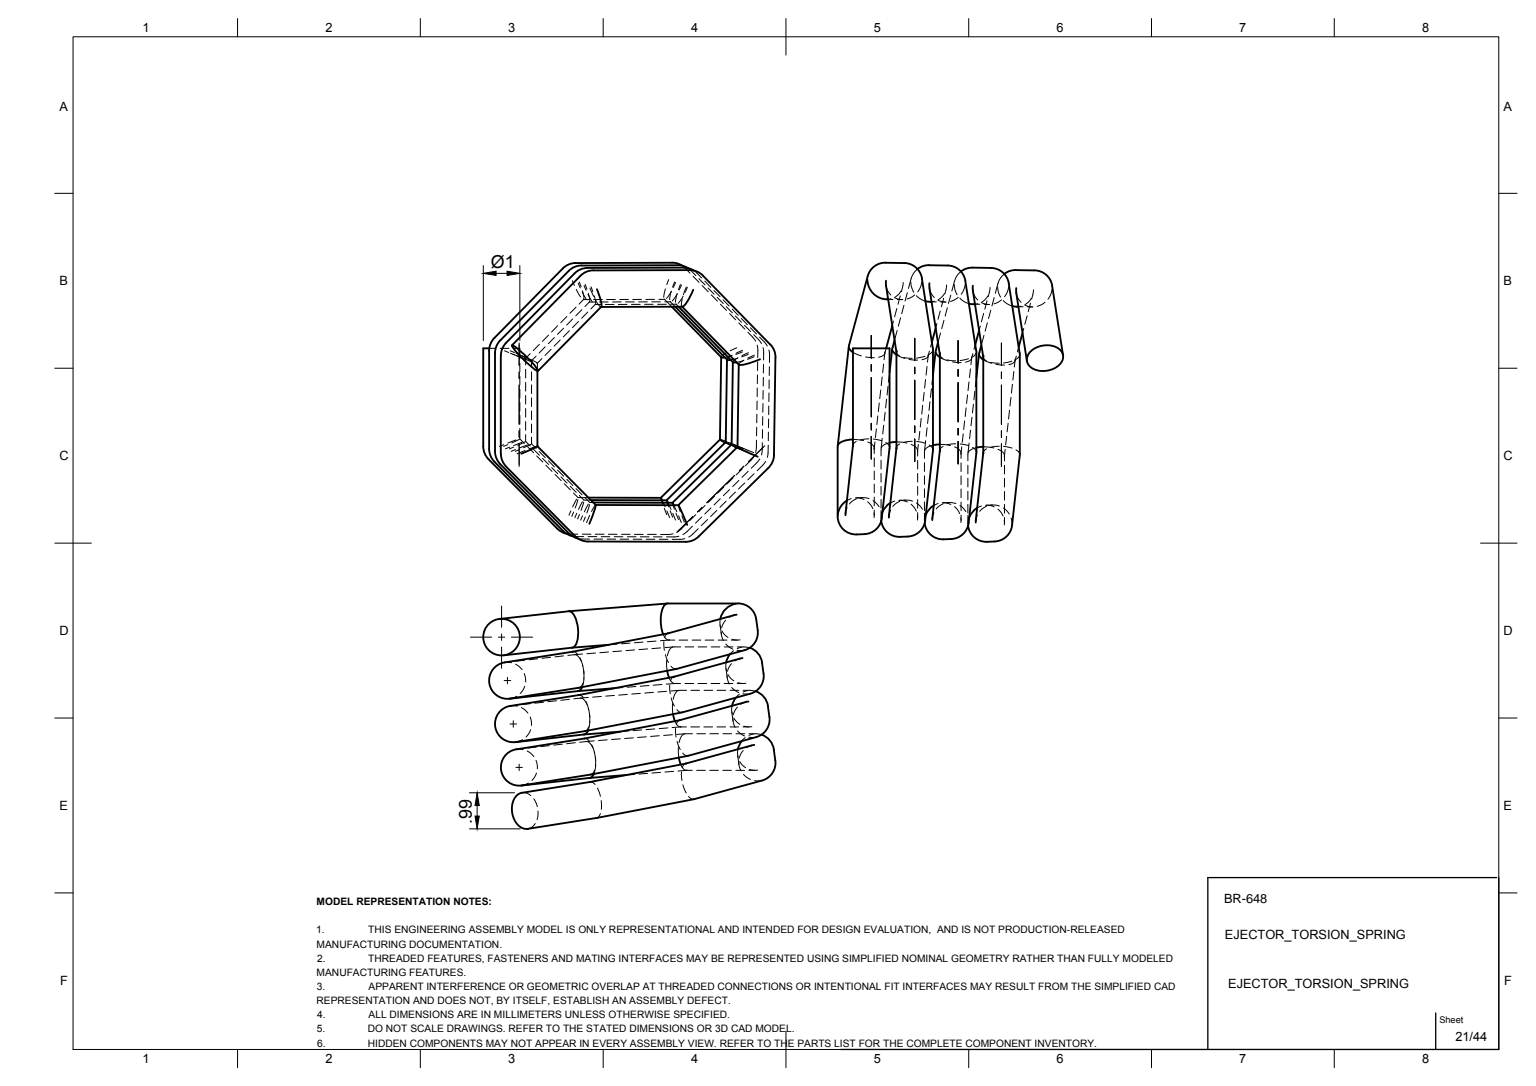
ISO-10303-21;
HEADER;
FILE_DESCRIPTION((''),'2;1');
FILE_NAME('EJECTOR_TORSION_SPRING.step','2026-10-01T22:05:39-07:00',(''),(''),'','','');
FILE_SCHEMA (('AUTOMOTIVE_DESIGN { 1 0 10303 214 3 1 1 }'));
ENDSEC;
DATA;
#10=MECHANICAL_DESIGN_GEOMETRIC_PRESENTATION_REPRESENTATION('',(#621),#24628);
#277=ELLIPSE('',#14403,0.0541051040647724,0.05) ;
#278=ELLIPSE('',#14404,0.0541051040647724,0.05) ;
#279=ELLIPSE('',#14405,0.0541051040647724,0.05) ;
#280=ELLIPSE('',#14408,0.0541051040647731,0.05) ;
#281=ELLIPSE('',#14409,0.0541051040647731,0.05) ;
#282=ELLIPSE('',#14411,0.0541051040647723,0.05) ;
#283=ELLIPSE('',#14413,0.0541051040647739,0.05) ;
#284=ELLIPSE('',#14415,0.0541051040647728,0.05) ;
#285=ELLIPSE('',#14417,0.0541051040647725,0.05) ;
#286=ELLIPSE('',#14418,0.0541051040647725,0.05) ;
#287=ELLIPSE('',#14420,0.0541051040647722,0.05) ;
#288=ELLIPSE('',#14421,0.0541051040647722,0.05) ;
#289=ELLIPSE('',#14422,0.0541051040647722,0.05) ;
#290=ELLIPSE('',#14424,0.0541051040647732,0.05) ;
#291=ELLIPSE('',#14425,0.0541051040647732,0.05) ;
#292=ELLIPSE('',#14427,0.054105104064773,0.05) ;
#293=ELLIPSE('',#14428,0.054105104064773,0.05) ;
#294=ELLIPSE('',#14429,0.054105104064773,0.05) ;
#295=ELLIPSE('',#14431,0.0541051040647731,0.05) ;
#296=ELLIPSE('',#14432,0.0541051040647731,0.05) ;
#297=ELLIPSE('',#14434,0.0541051040647723,0.05) ;
#298=ELLIPSE('',#14436,0.0541051040647739,0.05) ;
#299=ELLIPSE('',#14438,0.0541051040647728,0.05) ;
#300=ELLIPSE('',#14440,0.0541051040647725,0.05) ;
#301=ELLIPSE('',#14441,0.0541051040647725,0.05) ;
#302=ELLIPSE('',#14443,0.0541051040647722,0.05) ;
#303=ELLIPSE('',#14444,0.0541051040647722,0.05) ;
#304=ELLIPSE('',#14445,0.0541051040647722,0.05) ;
#305=ELLIPSE('',#14447,0.0541051040647732,0.05) ;
#306=ELLIPSE('',#14448,0.0541051040647732,0.05) ;
#307=ELLIPSE('',#14450,0.0541051040647732,0.05) ;
#308=ELLIPSE('',#14451,0.0541051040647732,0.05) ;
#309=ELLIPSE('',#14452,0.0541051040647732,0.05) ;
#310=ELLIPSE('',#14454,0.0541051040647731,0.05) ;
#311=ELLIPSE('',#14455,0.0541051040647731,0.05) ;
#312=ELLIPSE('',#14457,0.0541051040647721,0.05) ;
#313=ELLIPSE('',#14459,0.0541051040647739,0.05) ;
#314=ELLIPSE('',#14461,0.0541051040647728,0.05) ;
#315=ELLIPSE('',#14463,0.0541051040647725,0.05) ;
#316=ELLIPSE('',#14464,0.0541051040647725,0.05) ;
#317=ELLIPSE('',#14466,0.0541051040647719,0.05) ;
#318=ELLIPSE('',#14467,0.0541051040647719,0.05) ;
#319=ELLIPSE('',#14468,0.0541051040647719,0.05) ;
#320=ELLIPSE('',#14470,0.0541051040647732,0.05) ;
#321=ELLIPSE('',#14471,0.0541051040647732,0.05) ;
#322=ELLIPSE('',#14473,0.0541051040647732,0.05) ;
#323=ELLIPSE('',#14474,0.0541051040647732,0.05) ;
#324=ELLIPSE('',#14475,0.0541051040647732,0.05) ;
#325=ELLIPSE('',#14477,0.0541051040647731,0.05) ;
#326=ELLIPSE('',#14478,0.0541051040647731,0.05) ;
#327=ELLIPSE('',#14480,0.0541051040647723,0.05) ;
#328=ELLIPSE('',#14482,0.0541051040647732,0.05) ;
#329=ELLIPSE('',#14484,0.0541051040647732,0.05) ;
#330=ELLIPSE('',#14486,0.0541051040647725,0.05) ;
#331=ELLIPSE('',#14487,0.0541051040647725,0.05) ;
#332=ELLIPSE('',#14489,0.0541051040647719,0.05) ;
#333=ELLIPSE('',#14490,0.0541051040647719,0.05) ;
#334=ELLIPSE('',#14491,0.0541051040647719,0.05) ;
#359=SPHERICAL_SURFACE('',#14260,0.05) ;
#360=SPHERICAL_SURFACE('',#14263,0.05) ;
#361=SPHERICAL_SURFACE('',#14269,0.05) ;
#362=SPHERICAL_SURFACE('',#14274,0.05) ;
#363=SPHERICAL_SURFACE('',#14279,0.05) ;
#364=SPHERICAL_SURFACE('',#14284,0.05) ;
#365=SPHERICAL_SURFACE('',#14290,0.05) ;
#366=SPHERICAL_SURFACE('',#14293,0.05) ;
#367=SPHERICAL_SURFACE('',#14296,0.05) ;
#368=SPHERICAL_SURFACE('',#14299,0.05) ;
#369=SPHERICAL_SURFACE('',#14305,0.05) ;
#370=SPHERICAL_SURFACE('',#14310,0.05) ;
#371=SPHERICAL_SURFACE('',#14315,0.05) ;
#372=SPHERICAL_SURFACE('',#14320,0.05) ;
#373=SPHERICAL_SURFACE('',#14326,0.05) ;
#374=SPHERICAL_SURFACE('',#14329,0.05) ;
#375=SPHERICAL_SURFACE('',#14332,0.05) ;
#376=SPHERICAL_SURFACE('',#14335,0.05) ;
#377=SPHERICAL_SURFACE('',#14341,0.05) ;
#378=SPHERICAL_SURFACE('',#14346,0.05) ;
#379=SPHERICAL_SURFACE('',#14351,0.05) ;
#380=SPHERICAL_SURFACE('',#14356,0.05) ;
#381=SPHERICAL_SURFACE('',#14362,0.05) ;
#382=SPHERICAL_SURFACE('',#14365,0.05) ;
#383=SPHERICAL_SURFACE('',#14368,0.05) ;
#384=SPHERICAL_SURFACE('',#14371,0.05) ;
#385=SPHERICAL_SURFACE('',#14377,0.05) ;
#386=SPHERICAL_SURFACE('',#14382,0.05) ;
#387=SPHERICAL_SURFACE('',#14387,0.05) ;
#388=SPHERICAL_SURFACE('',#14392,0.05) ;
#389=SPHERICAL_SURFACE('',#14398,0.05) ;
#537=SHAPE_REPRESENTATION_RELATIONSHIP('SRR','None',#24809,#579) ;
#579=ADVANCED_BREP_SHAPE_REPRESENTATION('',(#661),#24599) ;
#621=STYLED_ITEM('',(#25030),#661) ;
#661=MANIFOLD_SOLID_BREP('EJECTOR_TORSION_SPRING',#13132) ;
#1356=LINE('',#21465,#2192) ;
#1357=LINE('',#21473,#2193) ;
#1358=LINE('',#21477,#2194) ;
#1359=LINE('',#21480,#2195) ;
#1360=LINE('',#21483,#2196) ;
#1361=LINE('',#21486,#2197) ;
#1362=LINE('',#21492,#2198) ;
#1363=LINE('',#21499,#2199) ;
#1364=LINE('',#21504,#2200) ;
#1365=LINE('',#21511,#2201) ;
#1366=LINE('',#21515,#2202) ;
#1367=LINE('',#21518,#2203) ;
#1368=LINE('',#21521,#2204) ;
#1369=LINE('',#21524,#2205) ;
#1370=LINE('',#21530,#2206) ;
#1371=LINE('',#21537,#2207) ;
#1372=LINE('',#21542,#2208) ;
#1373=LINE('',#21549,#2209) ;
#1374=LINE('',#21553,#2210) ;
#1375=LINE('',#21556,#2211) ;
#1376=LINE('',#21559,#2212) ;
#1377=LINE('',#21562,#2213) ;
#1378=LINE('',#21568,#2214) ;
#1379=LINE('',#21575,#2215) ;
#1380=LINE('',#21580,#2216) ;
#1381=LINE('',#21587,#2217) ;
#1382=LINE('',#21591,#2218) ;
#1383=LINE('',#21594,#2219) ;
#1384=LINE('',#21597,#2220) ;
#1385=LINE('',#21600,#2221) ;
#1386=LINE('',#21606,#2222) ;
#1387=LINE('',#21613,#2223) ;
#2192=VECTOR('',#17247,0.05) ;
#2193=VECTOR('',#17258,0.05) ;
#2194=VECTOR('',#17265,0.05) ;
#2195=VECTOR('',#17270,0.05) ;
#2196=VECTOR('',#17275,0.05) ;
#2197=VECTOR('',#17280,0.05) ;
#2198=VECTOR('',#17287,0.05) ;
#2199=VECTOR('',#17296,0.05) ;
#2200=VECTOR('',#17303,0.05) ;
#2201=VECTOR('',#17312,0.05) ;
#2202=VECTOR('',#17319,0.05) ;
#2203=VECTOR('',#17324,0.05) ;
#2204=VECTOR('',#17329,0.05) ;
#2205=VECTOR('',#17334,0.05) ;
#2206=VECTOR('',#17341,0.05) ;
#2207=VECTOR('',#17350,0.05) ;
#2208=VECTOR('',#17357,0.05) ;
#2209=VECTOR('',#17366,0.05) ;
#2210=VECTOR('',#17373,0.05) ;
#2211=VECTOR('',#17378,0.05) ;
#2212=VECTOR('',#17383,0.05) ;
#2213=VECTOR('',#17388,0.05) ;
#2214=VECTOR('',#17395,0.05) ;
#2215=VECTOR('',#17404,0.05) ;
#2216=VECTOR('',#17411,0.05) ;
#2217=VECTOR('',#17420,0.05) ;
#2218=VECTOR('',#17427,0.05) ;
#2219=VECTOR('',#17432,0.05) ;
#2220=VECTOR('',#17437,0.05) ;
#2221=VECTOR('',#17442,0.05) ;
#2222=VECTOR('',#17449,0.05) ;
#2223=VECTOR('',#17458,0.05) ;
#2812=CYLINDRICAL_SURFACE('',#14401,0.05) ;
#2813=CYLINDRICAL_SURFACE('',#14407,0.05) ;
#2814=CYLINDRICAL_SURFACE('',#14410,0.05) ;
#2815=CYLINDRICAL_SURFACE('',#14412,0.05) ;
#2816=CYLINDRICAL_SURFACE('',#14414,0.05) ;
#2817=CYLINDRICAL_SURFACE('',#14416,0.05) ;
#2818=CYLINDRICAL_SURFACE('',#14419,0.05) ;
#2819=CYLINDRICAL_SURFACE('',#14423,0.05) ;
#2820=CYLINDRICAL_SURFACE('',#14426,0.05) ;
#2821=CYLINDRICAL_SURFACE('',#14430,0.05) ;
#2822=CYLINDRICAL_SURFACE('',#14433,0.05) ;
#2823=CYLINDRICAL_SURFACE('',#14435,0.05) ;
#2824=CYLINDRICAL_SURFACE('',#14437,0.05) ;
#2825=CYLINDRICAL_SURFACE('',#14439,0.05) ;
#2826=CYLINDRICAL_SURFACE('',#14442,0.05) ;
#2827=CYLINDRICAL_SURFACE('',#14446,0.05) ;
#2828=CYLINDRICAL_SURFACE('',#14449,0.05) ;
#2829=CYLINDRICAL_SURFACE('',#14453,0.05) ;
#2830=CYLINDRICAL_SURFACE('',#14456,0.05) ;
#2831=CYLINDRICAL_SURFACE('',#14458,0.05) ;
#2832=CYLINDRICAL_SURFACE('',#14460,0.05) ;
#2833=CYLINDRICAL_SURFACE('',#14462,0.05) ;
#2834=CYLINDRICAL_SURFACE('',#14465,0.05) ;
#2835=CYLINDRICAL_SURFACE('',#14469,0.05) ;
#2836=CYLINDRICAL_SURFACE('',#14472,0.05) ;
#2837=CYLINDRICAL_SURFACE('',#14476,0.05) ;
#2838=CYLINDRICAL_SURFACE('',#14479,0.05) ;
#2839=CYLINDRICAL_SURFACE('',#14481,0.05) ;
#2840=CYLINDRICAL_SURFACE('',#14483,0.05) ;
#2841=CYLINDRICAL_SURFACE('',#14485,0.05) ;
#2842=CYLINDRICAL_SURFACE('',#14488,0.05) ;
#2843=CYLINDRICAL_SURFACE('',#14492,0.05) ;
#3244=FACE_OUTER_BOUND('',#4182,.T.) ;
#3245=FACE_OUTER_BOUND('',#4183,.T.) ;
#3246=FACE_OUTER_BOUND('',#4184,.T.) ;
#3247=FACE_OUTER_BOUND('',#4185,.T.) ;
#3248=FACE_OUTER_BOUND('',#4186,.T.) ;
#3249=FACE_OUTER_BOUND('',#4187,.T.) ;
#3250=FACE_OUTER_BOUND('',#4188,.T.) ;
#3251=FACE_OUTER_BOUND('',#4189,.T.) ;
#3252=FACE_OUTER_BOUND('',#4190,.T.) ;
#3253=FACE_OUTER_BOUND('',#4191,.T.) ;
#3254=FACE_OUTER_BOUND('',#4192,.T.) ;
#3255=FACE_OUTER_BOUND('',#4193,.T.) ;
#3256=FACE_OUTER_BOUND('',#4194,.T.) ;
#3257=FACE_OUTER_BOUND('',#4195,.T.) ;
#3258=FACE_OUTER_BOUND('',#4196,.T.) ;
#3259=FACE_OUTER_BOUND('',#4197,.T.) ;
#3260=FACE_OUTER_BOUND('',#4198,.T.) ;
#3261=FACE_OUTER_BOUND('',#4199,.T.) ;
#3262=FACE_OUTER_BOUND('',#4200,.T.) ;
#3263=FACE_OUTER_BOUND('',#4201,.T.) ;
#3264=FACE_OUTER_BOUND('',#4202,.T.) ;
#3265=FACE_OUTER_BOUND('',#4203,.T.) ;
#3266=FACE_OUTER_BOUND('',#4204,.T.) ;
#3267=FACE_OUTER_BOUND('',#4205,.T.) ;
#3268=FACE_OUTER_BOUND('',#4206,.T.) ;
#3269=FACE_OUTER_BOUND('',#4207,.T.) ;
#3270=FACE_OUTER_BOUND('',#4208,.T.) ;
#3271=FACE_OUTER_BOUND('',#4209,.T.) ;
#3272=FACE_OUTER_BOUND('',#4210,.T.) ;
#3273=FACE_OUTER_BOUND('',#4211,.T.) ;
#3274=FACE_OUTER_BOUND('',#4212,.T.) ;
#3275=FACE_OUTER_BOUND('',#4213,.T.) ;
#3276=FACE_OUTER_BOUND('',#4214,.T.) ;
#3277=FACE_OUTER_BOUND('',#4215,.T.) ;
#3278=FACE_OUTER_BOUND('',#4216,.T.) ;
#3279=FACE_OUTER_BOUND('',#4217,.T.) ;
#3280=FACE_OUTER_BOUND('',#4218,.T.) ;
#3281=FACE_OUTER_BOUND('',#4219,.T.) ;
#3282=FACE_OUTER_BOUND('',#4220,.T.) ;
#3283=FACE_OUTER_BOUND('',#4221,.T.) ;
#3284=FACE_OUTER_BOUND('',#4222,.T.) ;
#3285=FACE_OUTER_BOUND('',#4223,.T.) ;
#3286=FACE_OUTER_BOUND('',#4224,.T.) ;
#3287=FACE_OUTER_BOUND('',#4225,.T.) ;
#3288=FACE_OUTER_BOUND('',#4226,.T.) ;
#3289=FACE_OUTER_BOUND('',#4227,.T.) ;
#3290=FACE_OUTER_BOUND('',#4228,.T.) ;
#3291=FACE_OUTER_BOUND('',#4229,.T.) ;
#3292=FACE_OUTER_BOUND('',#4230,.T.) ;
#3293=FACE_OUTER_BOUND('',#4231,.T.) ;
#3294=FACE_OUTER_BOUND('',#4232,.T.) ;
#3295=FACE_OUTER_BOUND('',#4233,.T.) ;
#3296=FACE_OUTER_BOUND('',#4234,.T.) ;
#3297=FACE_OUTER_BOUND('',#4235,.T.) ;
#3298=FACE_OUTER_BOUND('',#4236,.T.) ;
#3299=FACE_OUTER_BOUND('',#4237,.T.) ;
#3300=FACE_OUTER_BOUND('',#4238,.T.) ;
#3301=FACE_OUTER_BOUND('',#4239,.T.) ;
#3302=FACE_OUTER_BOUND('',#4240,.T.) ;
#3303=FACE_OUTER_BOUND('',#4241,.T.) ;
#3304=FACE_OUTER_BOUND('',#4242,.T.) ;
#3305=FACE_OUTER_BOUND('',#4243,.T.) ;
#3306=FACE_OUTER_BOUND('',#4244,.T.) ;
#3307=FACE_OUTER_BOUND('',#4245,.T.) ;
#3308=FACE_OUTER_BOUND('',#4246,.T.) ;
#4182=EDGE_LOOP('',(#9801,#9802)) ;
#4183=EDGE_LOOP('',(#9803,#9804,#9805,#9806,#9807,#9808)) ;
#4184=EDGE_LOOP('',(#9809,#9810,#9811,#9812)) ;
#4185=EDGE_LOOP('',(#9813,#9814,#9815,#9816)) ;
#4186=EDGE_LOOP('',(#9817,#9818,#9819,#9820)) ;
#4187=EDGE_LOOP('',(#9821,#9822,#9823,#9824,#9825,#9826)) ;
#4188=EDGE_LOOP('',(#9827,#9828)) ;
#4189=EDGE_LOOP('',(#9829,#9830)) ;
#4190=EDGE_LOOP('',(#9831,#9832)) ;
#4191=EDGE_LOOP('',(#9833,#9834,#9835,#9836,#9837,#9838)) ;
#4192=EDGE_LOOP('',(#9839,#9840,#9841,#9842)) ;
#4193=EDGE_LOOP('',(#9843,#9844,#9845,#9846)) ;
#4194=EDGE_LOOP('',(#9847,#9848,#9849,#9850)) ;
#4195=EDGE_LOOP('',(#9851,#9852,#9853,#9854,#9855,#9856)) ;
#4196=EDGE_LOOP('',(#9857,#9858)) ;
#4197=EDGE_LOOP('',(#9859,#9860)) ;
#4198=EDGE_LOOP('',(#9861,#9862)) ;
#4199=EDGE_LOOP('',(#9863,#9864,#9865,#9866,#9867,#9868)) ;
#4200=EDGE_LOOP('',(#9869,#9870,#9871,#9872)) ;
#4201=EDGE_LOOP('',(#9873,#9874,#9875,#9876)) ;
#4202=EDGE_LOOP('',(#9877,#9878,#9879,#9880)) ;
#4203=EDGE_LOOP('',(#9881,#9882,#9883,#9884,#9885,#9886)) ;
#4204=EDGE_LOOP('',(#9887,#9888)) ;
#4205=EDGE_LOOP('',(#9889,#9890)) ;
#4206=EDGE_LOOP('',(#9891,#9892)) ;
#4207=EDGE_LOOP('',(#9893,#9894,#9895,#9896,#9897,#9898)) ;
#4208=EDGE_LOOP('',(#9899,#9900,#9901,#9902)) ;
#4209=EDGE_LOOP('',(#9903,#9904,#9905,#9906)) ;
#4210=EDGE_LOOP('',(#9907,#9908,#9909,#9910)) ;
#4211=EDGE_LOOP('',(#9911,#9912,#9913,#9914,#9915,#9916)) ;
#4212=EDGE_LOOP('',(#9917,#9918)) ;
#4213=EDGE_LOOP('',(#9919,#9920,#9921,#9922,#9923,#9924,#9925)) ;
#4214=EDGE_LOOP('',(#9926)) ;
#4215=EDGE_LOOP('',(#9927,#9928,#9929,#9930,#9931,#9932,#9933,#9934,#9935)) ;
#4216=EDGE_LOOP('',(#9936,#9937,#9938,#9939,#9940,#9941,#9942,#9943,#9944,
#9945)) ;
#4217=EDGE_LOOP('',(#9946,#9947,#9948,#9949,#9950,#9951,#9952,#9953)) ;
#4218=EDGE_LOOP('',(#9954,#9955,#9956,#9957,#9958,#9959,#9960,#9961)) ;
#4219=EDGE_LOOP('',(#9962,#9963,#9964,#9965,#9966,#9967,#9968,#9969,#9970,
#9971)) ;
#4220=EDGE_LOOP('',(#9972,#9973,#9974,#9975,#9976,#9977,#9978,#9979,#9980)) ;
#4221=EDGE_LOOP('',(#9981,#9982,#9983,#9984,#9985,#9986,#9987,#9988,#9989)) ;
#4222=EDGE_LOOP('',(#9990,#9991,#9992,#9993,#9994,#9995,#9996,#9997,#9998)) ;
#4223=EDGE_LOOP('',(#9999,#10000,#10001,#10002,#10003,#10004,#10005,#10006,
#10007)) ;
#4224=EDGE_LOOP('',(#10008,#10009,#10010,#10011,#10012,#10013,#10014,#10015,
#10016,#10017)) ;
#4225=EDGE_LOOP('',(#10018,#10019,#10020,#10021,#10022,#10023,#10024,#10025)) ;
#4226=EDGE_LOOP('',(#10026,#10027,#10028,#10029,#10030,#10031,#10032,#10033)) ;
#4227=EDGE_LOOP('',(#10034,#10035,#10036,#10037,#10038,#10039,#10040,#10041,
#10042,#10043)) ;
#4228=EDGE_LOOP('',(#10044,#10045,#10046,#10047,#10048,#10049,#10050,#10051,
#10052)) ;
#4229=EDGE_LOOP('',(#10053,#10054,#10055,#10056,#10057,#10058,#10059,#10060,
#10061)) ;
#4230=EDGE_LOOP('',(#10062,#10063,#10064,#10065,#10066,#10067,#10068,#10069,
#10070)) ;
#4231=EDGE_LOOP('',(#10071,#10072,#10073,#10074,#10075,#10076,#10077,#10078,
#10079)) ;
#4232=EDGE_LOOP('',(#10080,#10081,#10082,#10083,#10084,#10085,#10086,#10087,
#10088,#10089)) ;
#4233=EDGE_LOOP('',(#10090,#10091,#10092,#10093,#10094,#10095,#10096,#10097)) ;
#4234=EDGE_LOOP('',(#10098,#10099,#10100,#10101,#10102,#10103,#10104,#10105)) ;
#4235=EDGE_LOOP('',(#10106,#10107,#10108,#10109,#10110,#10111,#10112,#10113,
#10114,#10115)) ;
#4236=EDGE_LOOP('',(#10116,#10117,#10118,#10119,#10120,#10121,#10122,#10123,
#10124)) ;
#4237=EDGE_LOOP('',(#10125,#10126,#10127,#10128,#10129,#10130,#10131,#10132,
#10133)) ;
#4238=EDGE_LOOP('',(#10134,#10135,#10136,#10137,#10138,#10139,#10140,#10141,
#10142)) ;
#4239=EDGE_LOOP('',(#10143,#10144,#10145,#10146,#10147,#10148,#10149,#10150,
#10151)) ;
#4240=EDGE_LOOP('',(#10152,#10153,#10154,#10155,#10156,#10157,#10158,#10159,
#10160,#10161)) ;
#4241=EDGE_LOOP('',(#10162,#10163,#10164,#10165,#10166,#10167,#10168,#10169)) ;
#4242=EDGE_LOOP('',(#10170,#10171,#10172,#10173,#10174,#10175,#10176,#10177)) ;
#4243=EDGE_LOOP('',(#10178,#10179,#10180,#10181,#10182,#10183,#10184,#10185,
#10186,#10187)) ;
#4244=EDGE_LOOP('',(#10188,#10189,#10190,#10191,#10192,#10193,#10194,#10195,
#10196)) ;
#4245=EDGE_LOOP('',(#10197,#10198,#10199,#10200,#10201,#10202,#10203)) ;
#4246=EDGE_LOOP('',(#10204)) ;
#5048=CIRCLE('',#14261,0.05) ;
#5049=CIRCLE('',#14262,0.05) ;
#5050=CIRCLE('',#14264,0.05) ;
#5051=CIRCLE('',#14265,0.05) ;
#5052=CIRCLE('',#14266,0.05) ;
#5053=CIRCLE('',#14267,0.0499999999999998) ;
#5054=CIRCLE('',#14268,0.05) ;
#5055=CIRCLE('',#14270,0.05) ;
#5056=CIRCLE('',#14271,0.05) ;
#5057=CIRCLE('',#14272,0.05) ;
#5058=CIRCLE('',#14273,0.05) ;
#5059=CIRCLE('',#14275,0.05) ;
#5060=CIRCLE('',#14276,0.05) ;
#5061=CIRCLE('',#14277,0.05) ;
#5062=CIRCLE('',#14278,0.05) ;
#5063=CIRCLE('',#14280,0.05) ;
#5064=CIRCLE('',#14281,0.05) ;
#5065=CIRCLE('',#14282,0.05) ;
#5066=CIRCLE('',#14283,0.05) ;
#5067=CIRCLE('',#14285,0.05) ;
#5068=CIRCLE('',#14286,0.05) ;
#5069=CIRCLE('',#14287,0.0499999999999998) ;
#5070=CIRCLE('',#14288,0.05) ;
#5071=CIRCLE('',#14289,0.05) ;
#5072=CIRCLE('',#14291,0.05) ;
#5073=CIRCLE('',#14292,0.05) ;
#5074=CIRCLE('',#14294,0.05) ;
#5075=CIRCLE('',#14295,0.05) ;
#5076=CIRCLE('',#14297,0.05) ;
#5077=CIRCLE('',#14298,0.05) ;
#5078=CIRCLE('',#14300,0.05) ;
#5079=CIRCLE('',#14301,0.05) ;
#5080=CIRCLE('',#14302,0.05) ;
#5081=CIRCLE('',#14303,0.0499999999999998) ;
#5082=CIRCLE('',#14304,0.05) ;
#5083=CIRCLE('',#14306,0.05) ;
#5084=CIRCLE('',#14307,0.05) ;
#5085=CIRCLE('',#14308,0.05) ;
#5086=CIRCLE('',#14309,0.05) ;
#5087=CIRCLE('',#14311,0.05) ;
#5088=CIRCLE('',#14312,0.05) ;
#5089=CIRCLE('',#14313,0.05) ;
#5090=CIRCLE('',#14314,0.05) ;
#5091=CIRCLE('',#14316,0.05) ;
#5092=CIRCLE('',#14317,0.05) ;
#5093=CIRCLE('',#14318,0.05) ;
#5094=CIRCLE('',#14319,0.05) ;
#5095=CIRCLE('',#14321,0.05) ;
#5096=CIRCLE('',#14322,0.05) ;
#5097=CIRCLE('',#14323,0.0499999999999998) ;
#5098=CIRCLE('',#14324,0.05) ;
#5099=CIRCLE('',#14325,0.05) ;
#5100=CIRCLE('',#14327,0.05) ;
#5101=CIRCLE('',#14328,0.05) ;
#5102=CIRCLE('',#14330,0.05) ;
#5103=CIRCLE('',#14331,0.05) ;
#5104=CIRCLE('',#14333,0.05) ;
#5105=CIRCLE('',#14334,0.05) ;
#5106=CIRCLE('',#14336,0.05) ;
#5107=CIRCLE('',#14337,0.05) ;
#5108=CIRCLE('',#14338,0.05) ;
#5109=CIRCLE('',#14339,0.0499999999999998) ;
#5110=CIRCLE('',#14340,0.05) ;
#5111=CIRCLE('',#14342,0.05) ;
#5112=CIRCLE('',#14343,0.05) ;
#5113=CIRCLE('',#14344,0.05) ;
#5114=CIRCLE('',#14345,0.05) ;
#5115=CIRCLE('',#14347,0.05) ;
#5116=CIRCLE('',#14348,0.05) ;
#5117=CIRCLE('',#14349,0.05) ;
#5118=CIRCLE('',#14350,0.05) ;
#5119=CIRCLE('',#14352,0.05) ;
#5120=CIRCLE('',#14353,0.05) ;
#5121=CIRCLE('',#14354,0.05) ;
#5122=CIRCLE('',#14355,0.05) ;
#5123=CIRCLE('',#14357,0.05) ;
#5124=CIRCLE('',#14358,0.05) ;
#5125=CIRCLE('',#14359,0.0499999999999998) ;
#5126=CIRCLE('',#14360,0.05) ;
#5127=CIRCLE('',#14361,0.05) ;
#5128=CIRCLE('',#14363,0.05) ;
#5129=CIRCLE('',#14364,0.05) ;
#5130=CIRCLE('',#14366,0.05) ;
#5131=CIRCLE('',#14367,0.05) ;
#5132=CIRCLE('',#14369,0.05) ;
#5133=CIRCLE('',#14370,0.05) ;
#5134=CIRCLE('',#14372,0.05) ;
#5135=CIRCLE('',#14373,0.05) ;
#5136=CIRCLE('',#14374,0.05) ;
#5137=CIRCLE('',#14375,0.0499999999999998) ;
#5138=CIRCLE('',#14376,0.05) ;
#5139=CIRCLE('',#14378,0.05) ;
#5140=CIRCLE('',#14379,0.05) ;
#5141=CIRCLE('',#14380,0.05) ;
#5142=CIRCLE('',#14381,0.05) ;
#5143=CIRCLE('',#14383,0.05) ;
#5144=CIRCLE('',#14384,0.05) ;
#5145=CIRCLE('',#14385,0.05) ;
#5146=CIRCLE('',#14386,0.05) ;
#5147=CIRCLE('',#14388,0.05) ;
#5148=CIRCLE('',#14389,0.05) ;
#5149=CIRCLE('',#14390,0.05) ;
#5150=CIRCLE('',#14391,0.05) ;
#5151=CIRCLE('',#14393,0.05) ;
#5152=CIRCLE('',#14394,0.05) ;
#5153=CIRCLE('',#14395,0.0499999999999998) ;
#5154=CIRCLE('',#14396,0.05) ;
#5155=CIRCLE('',#14397,0.05) ;
#5156=CIRCLE('',#14399,0.05) ;
#5157=CIRCLE('',#14400,0.05) ;
#5158=CIRCLE('',#14402,0.05) ;
#5159=CIRCLE('',#14493,0.05) ;
#5975=VERTEX_POINT('',#21211) ;
#5976=VERTEX_POINT('',#21212) ;
#5977=VERTEX_POINT('',#21216) ;
#5978=VERTEX_POINT('',#21217) ;
#5979=VERTEX_POINT('',#21219) ;
#5980=VERTEX_POINT('',#21221) ;
#5981=VERTEX_POINT('',#21223) ;
#5982=VERTEX_POINT('',#21227) ;
#5983=VERTEX_POINT('',#21228) ;
#5984=VERTEX_POINT('',#21230) ;
#5985=VERTEX_POINT('',#21232) ;
#5986=VERTEX_POINT('',#21236) ;
#5987=VERTEX_POINT('',#21237) ;
#5988=VERTEX_POINT('',#21239) ;
#5989=VERTEX_POINT('',#21241) ;
#5990=VERTEX_POINT('',#21245) ;
#5991=VERTEX_POINT('',#21246) ;
#5992=VERTEX_POINT('',#21248) ;
#5993=VERTEX_POINT('',#21250) ;
#5994=VERTEX_POINT('',#21254) ;
#5995=VERTEX_POINT('',#21255) ;
#5996=VERTEX_POINT('',#21257) ;
#5997=VERTEX_POINT('',#21259) ;
#5998=VERTEX_POINT('',#21261) ;
#5999=VERTEX_POINT('',#21265) ;
#6000=VERTEX_POINT('',#21266) ;
#6001=VERTEX_POINT('',#21270) ;
#6002=VERTEX_POINT('',#21271) ;
#6003=VERTEX_POINT('',#21275) ;
#6004=VERTEX_POINT('',#21276) ;
#6005=VERTEX_POINT('',#21280) ;
#6006=VERTEX_POINT('',#21281) ;
#6007=VERTEX_POINT('',#21283) ;
#6008=VERTEX_POINT('',#21285) ;
#6009=VERTEX_POINT('',#21287) ;
#6010=VERTEX_POINT('',#21291) ;
#6011=VERTEX_POINT('',#21292) ;
#6012=VERTEX_POINT('',#21294) ;
#6013=VERTEX_POINT('',#21296) ;
#6014=VERTEX_POINT('',#21300) ;
#6015=VERTEX_POINT('',#21301) ;
#6016=VERTEX_POINT('',#21303) ;
#6017=VERTEX_POINT('',#21305) ;
#6018=VERTEX_POINT('',#21309) ;
#6019=VERTEX_POINT('',#21310) ;
#6020=VERTEX_POINT('',#21312) ;
#6021=VERTEX_POINT('',#21314) ;
#6022=VERTEX_POINT('',#21318) ;
#6023=VERTEX_POINT('',#21319) ;
#6024=VERTEX_POINT('',#21321) ;
#6025=VERTEX_POINT('',#21323) ;
#6026=VERTEX_POINT('',#21325) ;
#6027=VERTEX_POINT('',#21329) ;
#6028=VERTEX_POINT('',#21330) ;
#6029=VERTEX_POINT('',#21334) ;
#6030=VERTEX_POINT('',#21335) ;
#6031=VERTEX_POINT('',#21339) ;
#6032=VERTEX_POINT('',#21340) ;
#6033=VERTEX_POINT('',#21344) ;
#6034=VERTEX_POINT('',#21345) ;
#6035=VERTEX_POINT('',#21347) ;
#6036=VERTEX_POINT('',#21349) ;
#6037=VERTEX_POINT('',#21351) ;
#6038=VERTEX_POINT('',#21355) ;
#6039=VERTEX_POINT('',#21356) ;
#6040=VERTEX_POINT('',#21358) ;
#6041=VERTEX_POINT('',#21360) ;
#6042=VERTEX_POINT('',#21364) ;
#6043=VERTEX_POINT('',#21365) ;
#6044=VERTEX_POINT('',#21367) ;
#6045=VERTEX_POINT('',#21369) ;
#6046=VERTEX_POINT('',#21373) ;
#6047=VERTEX_POINT('',#21374) ;
#6048=VERTEX_POINT('',#21376) ;
#6049=VERTEX_POINT('',#21378) ;
#6050=VERTEX_POINT('',#21382) ;
#6051=VERTEX_POINT('',#21383) ;
#6052=VERTEX_POINT('',#21385) ;
#6053=VERTEX_POINT('',#21387) ;
#6054=VERTEX_POINT('',#21389) ;
#6055=VERTEX_POINT('',#21393) ;
#6056=VERTEX_POINT('',#21394) ;
#6057=VERTEX_POINT('',#21398) ;
#6058=VERTEX_POINT('',#21399) ;
#6059=VERTEX_POINT('',#21403) ;
#6060=VERTEX_POINT('',#21404) ;
#6061=VERTEX_POINT('',#21408) ;
#6062=VERTEX_POINT('',#21409) ;
#6063=VERTEX_POINT('',#21411) ;
#6064=VERTEX_POINT('',#21413) ;
#6065=VERTEX_POINT('',#21415) ;
#6066=VERTEX_POINT('',#21419) ;
#6067=VERTEX_POINT('',#21420) ;
#6068=VERTEX_POINT('',#21422) ;
#6069=VERTEX_POINT('',#21424) ;
#6070=VERTEX_POINT('',#21428) ;
#6071=VERTEX_POINT('',#21429) ;
#6072=VERTEX_POINT('',#21431) ;
#6073=VERTEX_POINT('',#21433) ;
#6074=VERTEX_POINT('',#21437) ;
#6075=VERTEX_POINT('',#21438) ;
#6076=VERTEX_POINT('',#21440) ;
#6077=VERTEX_POINT('',#21442) ;
#6078=VERTEX_POINT('',#21446) ;
#6079=VERTEX_POINT('',#21447) ;
#6080=VERTEX_POINT('',#21449) ;
#6081=VERTEX_POINT('',#21451) ;
#6082=VERTEX_POINT('',#21453) ;
#6083=VERTEX_POINT('',#21457) ;
#6084=VERTEX_POINT('',#21458) ;
#6085=VERTEX_POINT('',#21462) ;
#6086=VERTEX_POINT('',#21464) ;
#6087=VERTEX_POINT('',#21466) ;
#6088=VERTEX_POINT('',#21472) ;
#6089=VERTEX_POINT('',#21487) ;
#6090=VERTEX_POINT('',#21491) ;
#6091=VERTEX_POINT('',#21493) ;
#6092=VERTEX_POINT('',#21498) ;
#6093=VERTEX_POINT('',#21503) ;
#6094=VERTEX_POINT('',#21505) ;
#6095=VERTEX_POINT('',#21510) ;
#6096=VERTEX_POINT('',#21525) ;
#6097=VERTEX_POINT('',#21529) ;
#6098=VERTEX_POINT('',#21531) ;
#6099=VERTEX_POINT('',#21536) ;
#6100=VERTEX_POINT('',#21541) ;
#6101=VERTEX_POINT('',#21543) ;
#6102=VERTEX_POINT('',#21548) ;
#6103=VERTEX_POINT('',#21563) ;
#6104=VERTEX_POINT('',#21567) ;
#6105=VERTEX_POINT('',#21569) ;
#6106=VERTEX_POINT('',#21574) ;
#6107=VERTEX_POINT('',#21579) ;
#6108=VERTEX_POINT('',#21581) ;
#6109=VERTEX_POINT('',#21586) ;
#6110=VERTEX_POINT('',#21601) ;
#6111=VERTEX_POINT('',#21605) ;
#6112=VERTEX_POINT('',#21607) ;
#6113=VERTEX_POINT('',#21612) ;
#7390=EDGE_CURVE('',#5975,#5976,#5048,.T.) ;
#7391=EDGE_CURVE('',#5976,#5975,#5049,.T.) ;
#7392=EDGE_CURVE('',#5977,#5978,#5050,.T.) ;
#7393=EDGE_CURVE('',#5978,#5979,#5051,.T.) ;
#7394=EDGE_CURVE('',#5979,#5980,#5052,.T.) ;
#7395=EDGE_CURVE('',#5981,#5980,#5053,.T.) ;
#7396=EDGE_CURVE('',#5980,#5977,#5054,.T.) ;
#7397=EDGE_CURVE('',#5982,#5983,#5055,.T.) ;
#7398=EDGE_CURVE('',#5983,#5984,#5056,.T.) ;
#7399=EDGE_CURVE('',#5984,#5985,#5057,.T.) ;
#7400=EDGE_CURVE('',#5985,#5982,#5058,.T.) ;
#7401=EDGE_CURVE('',#5986,#5987,#5059,.T.) ;
#7402=EDGE_CURVE('',#5987,#5988,#5060,.T.) ;
#7403=EDGE_CURVE('',#5988,#5989,#5061,.T.) ;
#7404=EDGE_CURVE('',#5989,#5986,#5062,.T.) ;
#7405=EDGE_CURVE('',#5990,#5991,#5063,.T.) ;
#7406=EDGE_CURVE('',#5991,#5992,#5064,.T.) ;
#7407=EDGE_CURVE('',#5992,#5993,#5065,.T.) ;
#7408=EDGE_CURVE('',#5993,#5990,#5066,.T.) ;
#7409=EDGE_CURVE('',#5994,#5995,#5067,.T.) ;
#7410=EDGE_CURVE('',#5995,#5996,#5068,.T.) ;
#7411=EDGE_CURVE('',#5996,#5997,#5069,.T.) ;
#7412=EDGE_CURVE('',#5996,#5998,#5070,.T.) ;
#7413=EDGE_CURVE('',#5998,#5994,#5071,.T.) ;
#7414=EDGE_CURVE('',#5999,#6000,#5072,.T.) ;
#7415=EDGE_CURVE('',#6000,#5999,#5073,.T.) ;
#7416=EDGE_CURVE('',#6001,#6002,#5074,.T.) ;
#7417=EDGE_CURVE('',#6002,#6001,#5075,.T.) ;
#7418=EDGE_CURVE('',#6003,#6004,#5076,.T.) ;
#7419=EDGE_CURVE('',#6004,#6003,#5077,.T.) ;
#7420=EDGE_CURVE('',#6005,#6006,#5078,.T.) ;
#7421=EDGE_CURVE('',#6006,#6007,#5079,.T.) ;
#7422=EDGE_CURVE('',#6007,#6008,#5080,.T.) ;
#7423=EDGE_CURVE('',#6009,#6008,#5081,.T.) ;
#7424=EDGE_CURVE('',#6008,#6005,#5082,.T.) ;
#7425=EDGE_CURVE('',#6010,#6011,#5083,.T.) ;
#7426=EDGE_CURVE('',#6011,#6012,#5084,.T.) ;
#7427=EDGE_CURVE('',#6012,#6013,#5085,.T.) ;
#7428=EDGE_CURVE('',#6013,#6010,#5086,.T.) ;
#7429=EDGE_CURVE('',#6014,#6015,#5087,.T.) ;
#7430=EDGE_CURVE('',#6015,#6016,#5088,.T.) ;
#7431=EDGE_CURVE('',#6016,#6017,#5089,.T.) ;
#7432=EDGE_CURVE('',#6017,#6014,#5090,.T.) ;
#7433=EDGE_CURVE('',#6018,#6019,#5091,.T.) ;
#7434=EDGE_CURVE('',#6019,#6020,#5092,.T.) ;
#7435=EDGE_CURVE('',#6020,#6021,#5093,.T.) ;
#7436=EDGE_CURVE('',#6021,#6018,#5094,.T.) ;
#7437=EDGE_CURVE('',#6022,#6023,#5095,.T.) ;
#7438=EDGE_CURVE('',#6023,#6024,#5096,.T.) ;
#7439=EDGE_CURVE('',#6024,#6025,#5097,.T.) ;
#7440=EDGE_CURVE('',#6024,#6026,#5098,.T.) ;
#7441=EDGE_CURVE('',#6026,#6022,#5099,.T.) ;
#7442=EDGE_CURVE('',#6027,#6028,#5100,.T.) ;
#7443=EDGE_CURVE('',#6028,#6027,#5101,.T.) ;
#7444=EDGE_CURVE('',#6029,#6030,#5102,.T.) ;
#7445=EDGE_CURVE('',#6030,#6029,#5103,.T.) ;
#7446=EDGE_CURVE('',#6031,#6032,#5104,.T.) ;
#7447=EDGE_CURVE('',#6032,#6031,#5105,.T.) ;
#7448=EDGE_CURVE('',#6033,#6034,#5106,.T.) ;
#7449=EDGE_CURVE('',#6034,#6035,#5107,.T.) ;
#7450=EDGE_CURVE('',#6035,#6036,#5108,.T.) ;
#7451=EDGE_CURVE('',#6037,#6036,#5109,.T.) ;
#7452=EDGE_CURVE('',#6036,#6033,#5110,.T.) ;
#7453=EDGE_CURVE('',#6038,#6039,#5111,.T.) ;
#7454=EDGE_CURVE('',#6039,#6040,#5112,.T.) ;
#7455=EDGE_CURVE('',#6040,#6041,#5113,.T.) ;
#7456=EDGE_CURVE('',#6041,#6038,#5114,.T.) ;
#7457=EDGE_CURVE('',#6042,#6043,#5115,.T.) ;
#7458=EDGE_CURVE('',#6043,#6044,#5116,.T.) ;
#7459=EDGE_CURVE('',#6044,#6045,#5117,.T.) ;
#7460=EDGE_CURVE('',#6045,#6042,#5118,.T.) ;
#7461=EDGE_CURVE('',#6046,#6047,#5119,.T.) ;
#7462=EDGE_CURVE('',#6047,#6048,#5120,.T.) ;
#7463=EDGE_CURVE('',#6048,#6049,#5121,.T.) ;
#7464=EDGE_CURVE('',#6049,#6046,#5122,.T.) ;
#7465=EDGE_CURVE('',#6050,#6051,#5123,.T.) ;
#7466=EDGE_CURVE('',#6051,#6052,#5124,.T.) ;
#7467=EDGE_CURVE('',#6052,#6053,#5125,.T.) ;
#7468=EDGE_CURVE('',#6052,#6054,#5126,.T.) ;
#7469=EDGE_CURVE('',#6054,#6050,#5127,.T.) ;
#7470=EDGE_CURVE('',#6055,#6056,#5128,.T.) ;
#7471=EDGE_CURVE('',#6056,#6055,#5129,.T.) ;
#7472=EDGE_CURVE('',#6057,#6058,#5130,.T.) ;
#7473=EDGE_CURVE('',#6058,#6057,#5131,.T.) ;
#7474=EDGE_CURVE('',#6059,#6060,#5132,.T.) ;
#7475=EDGE_CURVE('',#6060,#6059,#5133,.T.) ;
#7476=EDGE_CURVE('',#6061,#6062,#5134,.T.) ;
#7477=EDGE_CURVE('',#6062,#6063,#5135,.T.) ;
#7478=EDGE_CURVE('',#6063,#6064,#5136,.T.) ;
#7479=EDGE_CURVE('',#6065,#6064,#5137,.T.) ;
#7480=EDGE_CURVE('',#6064,#6061,#5138,.T.) ;
#7481=EDGE_CURVE('',#6066,#6067,#5139,.T.) ;
#7482=EDGE_CURVE('',#6067,#6068,#5140,.T.) ;
#7483=EDGE_CURVE('',#6068,#6069,#5141,.T.) ;
#7484=EDGE_CURVE('',#6069,#6066,#5142,.T.) ;
#7485=EDGE_CURVE('',#6070,#6071,#5143,.T.) ;
#7486=EDGE_CURVE('',#6071,#6072,#5144,.T.) ;
#7487=EDGE_CURVE('',#6072,#6073,#5145,.T.) ;
#7488=EDGE_CURVE('',#6073,#6070,#5146,.T.) ;
#7489=EDGE_CURVE('',#6074,#6075,#5147,.T.) ;
#7490=EDGE_CURVE('',#6075,#6076,#5148,.T.) ;
#7491=EDGE_CURVE('',#6076,#6077,#5149,.T.) ;
#7492=EDGE_CURVE('',#6077,#6074,#5150,.T.) ;
#7493=EDGE_CURVE('',#6078,#6079,#5151,.T.) ;
#7494=EDGE_CURVE('',#6079,#6080,#5152,.T.) ;
#7495=EDGE_CURVE('',#6080,#6081,#5153,.T.) ;
#7496=EDGE_CURVE('',#6080,#6082,#5154,.T.) ;
#7497=EDGE_CURVE('',#6082,#6078,#5155,.T.) ;
#7498=EDGE_CURVE('',#6083,#6084,#5156,.T.) ;
#7499=EDGE_CURVE('',#6084,#6083,#5157,.T.) ;
#7500=EDGE_CURVE('',#6085,#6085,#5158,.T.) ;
#7501=EDGE_CURVE('',#6085,#6086,#1356,.T.) ;
#7502=EDGE_CURVE('',#6087,#6086,#277,.T.) ;
#7503=EDGE_CURVE('',#5976,#6087,#278,.T.) ;
#7504=EDGE_CURVE('',#6086,#5975,#279,.T.) ;
#7505=EDGE_CURVE('',#6087,#6088,#1357,.T.) ;
#7506=EDGE_CURVE('',#5978,#6088,#280,.T.) ;
#7507=EDGE_CURVE('',#6088,#5977,#281,.T.) ;
#7508=EDGE_CURVE('',#5979,#5983,#1358,.T.) ;
#7509=EDGE_CURVE('',#5984,#5982,#282,.T.) ;
#7510=EDGE_CURVE('',#5985,#5987,#1359,.T.) ;
#7511=EDGE_CURVE('',#5988,#5986,#283,.T.) ;
#7512=EDGE_CURVE('',#5989,#5991,#1360,.T.) ;
#7513=EDGE_CURVE('',#5992,#5990,#284,.T.) ;
#7514=EDGE_CURVE('',#5993,#5995,#1361,.T.) ;
#7515=EDGE_CURVE('',#6089,#5994,#285,.T.) ;
#7516=EDGE_CURVE('',#5998,#6089,#286,.T.) ;
#7517=EDGE_CURVE('',#6089,#6090,#1362,.T.) ;
#7518=EDGE_CURVE('',#6091,#6090,#287,.T.) ;
#7519=EDGE_CURVE('',#6000,#6091,#288,.T.) ;
#7520=EDGE_CURVE('',#6090,#5999,#289,.T.) ;
#7521=EDGE_CURVE('',#6091,#6092,#1363,.T.) ;
#7522=EDGE_CURVE('',#6002,#6092,#290,.T.) ;
#7523=EDGE_CURVE('',#6092,#6001,#291,.T.) ;
#7524=EDGE_CURVE('',#6092,#6093,#1364,.T.) ;
#7525=EDGE_CURVE('',#6094,#6093,#292,.T.) ;
#7526=EDGE_CURVE('',#6004,#6094,#293,.T.) ;
#7527=EDGE_CURVE('',#6093,#6003,#294,.T.) ;
#7528=EDGE_CURVE('',#6094,#6095,#1365,.T.) ;
#7529=EDGE_CURVE('',#6006,#6095,#295,.T.) ;
#7530=EDGE_CURVE('',#6095,#6005,#296,.T.) ;
#7531=EDGE_CURVE('',#6007,#6011,#1366,.T.) ;
#7532=EDGE_CURVE('',#6012,#6010,#297,.T.) ;
#7533=EDGE_CURVE('',#6013,#6015,#1367,.T.) ;
#7534=EDGE_CURVE('',#6016,#6014,#298,.T.) ;
#7535=EDGE_CURVE('',#6017,#6019,#1368,.T.) ;
#7536=EDGE_CURVE('',#6020,#6018,#299,.T.) ;
#7537=EDGE_CURVE('',#6021,#6023,#1369,.T.) ;
#7538=EDGE_CURVE('',#6096,#6022,#300,.T.) ;
#7539=EDGE_CURVE('',#6026,#6096,#301,.T.) ;
#7540=EDGE_CURVE('',#6096,#6097,#1370,.T.) ;
#7541=EDGE_CURVE('',#6098,#6097,#302,.T.) ;
#7542=EDGE_CURVE('',#6028,#6098,#303,.T.) ;
#7543=EDGE_CURVE('',#6097,#6027,#304,.T.) ;
#7544=EDGE_CURVE('',#6098,#6099,#1371,.T.) ;
#7545=EDGE_CURVE('',#6030,#6099,#305,.T.) ;
#7546=EDGE_CURVE('',#6099,#6029,#306,.T.) ;
#7547=EDGE_CURVE('',#6099,#6100,#1372,.T.) ;
#7548=EDGE_CURVE('',#6101,#6100,#307,.T.) ;
#7549=EDGE_CURVE('',#6032,#6101,#308,.T.) ;
#7550=EDGE_CURVE('',#6100,#6031,#309,.T.) ;
#7551=EDGE_CURVE('',#6101,#6102,#1373,.T.) ;
#7552=EDGE_CURVE('',#6034,#6102,#310,.T.) ;
#7553=EDGE_CURVE('',#6102,#6033,#311,.T.) ;
#7554=EDGE_CURVE('',#6035,#6039,#1374,.T.) ;
#7555=EDGE_CURVE('',#6040,#6038,#312,.T.) ;
#7556=EDGE_CURVE('',#6041,#6043,#1375,.T.) ;
#7557=EDGE_CURVE('',#6044,#6042,#313,.T.) ;
#7558=EDGE_CURVE('',#6045,#6047,#1376,.T.) ;
#7559=EDGE_CURVE('',#6048,#6046,#314,.T.) ;
#7560=EDGE_CURVE('',#6049,#6051,#1377,.T.) ;
#7561=EDGE_CURVE('',#6103,#6050,#315,.T.) ;
#7562=EDGE_CURVE('',#6054,#6103,#316,.T.) ;
#7563=EDGE_CURVE('',#6103,#6104,#1378,.T.) ;
#7564=EDGE_CURVE('',#6105,#6104,#317,.T.) ;
#7565=EDGE_CURVE('',#6056,#6105,#318,.T.) ;
#7566=EDGE_CURVE('',#6104,#6055,#319,.T.) ;
#7567=EDGE_CURVE('',#6105,#6106,#1379,.T.) ;
#7568=EDGE_CURVE('',#6058,#6106,#320,.T.) ;
#7569=EDGE_CURVE('',#6106,#6057,#321,.T.) ;
#7570=EDGE_CURVE('',#6106,#6107,#1380,.T.) ;
#7571=EDGE_CURVE('',#6108,#6107,#322,.T.) ;
#7572=EDGE_CURVE('',#6060,#6108,#323,.T.) ;
#7573=EDGE_CURVE('',#6107,#6059,#324,.T.) ;
#7574=EDGE_CURVE('',#6108,#6109,#1381,.T.) ;
#7575=EDGE_CURVE('',#6062,#6109,#325,.T.) ;
#7576=EDGE_CURVE('',#6109,#6061,#326,.T.) ;
#7577=EDGE_CURVE('',#6063,#6067,#1382,.T.) ;
#7578=EDGE_CURVE('',#6068,#6066,#327,.T.) ;
#7579=EDGE_CURVE('',#6069,#6071,#1383,.T.) ;
#7580=EDGE_CURVE('',#6072,#6070,#328,.T.) ;
#7581=EDGE_CURVE('',#6073,#6075,#1384,.T.) ;
#7582=EDGE_CURVE('',#6076,#6074,#329,.T.) ;
#7583=EDGE_CURVE('',#6077,#6079,#1385,.T.) ;
#7584=EDGE_CURVE('',#6110,#6078,#330,.T.) ;
#7585=EDGE_CURVE('',#6082,#6110,#331,.T.) ;
#7586=EDGE_CURVE('',#6110,#6111,#1386,.T.) ;
#7587=EDGE_CURVE('',#6112,#6111,#332,.T.) ;
#7588=EDGE_CURVE('',#6084,#6112,#333,.T.) ;
#7589=EDGE_CURVE('',#6111,#6083,#334,.T.) ;
#7590=EDGE_CURVE('',#6112,#6113,#1387,.T.) ;
#7591=EDGE_CURVE('',#6113,#6113,#5159,.T.) ;
#9801=ORIENTED_EDGE('',*,*,#7390,.T.) ;
#9802=ORIENTED_EDGE('',*,*,#7391,.T.) ;
#9803=ORIENTED_EDGE('',*,*,#7392,.T.) ;
#9804=ORIENTED_EDGE('',*,*,#7393,.T.) ;
#9805=ORIENTED_EDGE('',*,*,#7394,.T.) ;
#9806=ORIENTED_EDGE('',*,*,#7395,.F.) ;
#9807=ORIENTED_EDGE('',*,*,#7395,.T.) ;
#9808=ORIENTED_EDGE('',*,*,#7396,.T.) ;
#9809=ORIENTED_EDGE('',*,*,#7397,.T.) ;
#9810=ORIENTED_EDGE('',*,*,#7398,.T.) ;
#9811=ORIENTED_EDGE('',*,*,#7399,.T.) ;
#9812=ORIENTED_EDGE('',*,*,#7400,.T.) ;
#9813=ORIENTED_EDGE('',*,*,#7401,.T.) ;
#9814=ORIENTED_EDGE('',*,*,#7402,.T.) ;
#9815=ORIENTED_EDGE('',*,*,#7403,.T.) ;
#9816=ORIENTED_EDGE('',*,*,#7404,.T.) ;
#9817=ORIENTED_EDGE('',*,*,#7405,.T.) ;
#9818=ORIENTED_EDGE('',*,*,#7406,.T.) ;
#9819=ORIENTED_EDGE('',*,*,#7407,.T.) ;
#9820=ORIENTED_EDGE('',*,*,#7408,.T.) ;
#9821=ORIENTED_EDGE('',*,*,#7409,.T.) ;
#9822=ORIENTED_EDGE('',*,*,#7410,.T.) ;
#9823=ORIENTED_EDGE('',*,*,#7411,.T.) ;
#9824=ORIENTED_EDGE('',*,*,#7411,.F.) ;
#9825=ORIENTED_EDGE('',*,*,#7412,.T.) ;
#9826=ORIENTED_EDGE('',*,*,#7413,.T.) ;
#9827=ORIENTED_EDGE('',*,*,#7414,.T.) ;
#9828=ORIENTED_EDGE('',*,*,#7415,.T.) ;
#9829=ORIENTED_EDGE('',*,*,#7416,.T.) ;
#9830=ORIENTED_EDGE('',*,*,#7417,.T.) ;
#9831=ORIENTED_EDGE('',*,*,#7418,.T.) ;
#9832=ORIENTED_EDGE('',*,*,#7419,.T.) ;
#9833=ORIENTED_EDGE('',*,*,#7420,.T.) ;
#9834=ORIENTED_EDGE('',*,*,#7421,.T.) ;
#9835=ORIENTED_EDGE('',*,*,#7422,.T.) ;
#9836=ORIENTED_EDGE('',*,*,#7423,.F.) ;
#9837=ORIENTED_EDGE('',*,*,#7423,.T.) ;
#9838=ORIENTED_EDGE('',*,*,#7424,.T.) ;
#9839=ORIENTED_EDGE('',*,*,#7425,.T.) ;
#9840=ORIENTED_EDGE('',*,*,#7426,.T.) ;
#9841=ORIENTED_EDGE('',*,*,#7427,.T.) ;
#9842=ORIENTED_EDGE('',*,*,#7428,.T.) ;
#9843=ORIENTED_EDGE('',*,*,#7429,.T.) ;
#9844=ORIENTED_EDGE('',*,*,#7430,.T.) ;
#9845=ORIENTED_EDGE('',*,*,#7431,.T.) ;
#9846=ORIENTED_EDGE('',*,*,#7432,.T.) ;
#9847=ORIENTED_EDGE('',*,*,#7433,.T.) ;
#9848=ORIENTED_EDGE('',*,*,#7434,.T.) ;
#9849=ORIENTED_EDGE('',*,*,#7435,.T.) ;
#9850=ORIENTED_EDGE('',*,*,#7436,.T.) ;
#9851=ORIENTED_EDGE('',*,*,#7437,.T.) ;
#9852=ORIENTED_EDGE('',*,*,#7438,.T.) ;
#9853=ORIENTED_EDGE('',*,*,#7439,.T.) ;
#9854=ORIENTED_EDGE('',*,*,#7439,.F.) ;
#9855=ORIENTED_EDGE('',*,*,#7440,.T.) ;
#9856=ORIENTED_EDGE('',*,*,#7441,.T.) ;
#9857=ORIENTED_EDGE('',*,*,#7442,.T.) ;
#9858=ORIENTED_EDGE('',*,*,#7443,.T.) ;
#9859=ORIENTED_EDGE('',*,*,#7444,.T.) ;
#9860=ORIENTED_EDGE('',*,*,#7445,.T.) ;
#9861=ORIENTED_EDGE('',*,*,#7446,.T.) ;
#9862=ORIENTED_EDGE('',*,*,#7447,.T.) ;
#9863=ORIENTED_EDGE('',*,*,#7448,.T.) ;
#9864=ORIENTED_EDGE('',*,*,#7449,.T.) ;
#9865=ORIENTED_EDGE('',*,*,#7450,.T.) ;
#9866=ORIENTED_EDGE('',*,*,#7451,.F.) ;
#9867=ORIENTED_EDGE('',*,*,#7451,.T.) ;
#9868=ORIENTED_EDGE('',*,*,#7452,.T.) ;
#9869=ORIENTED_EDGE('',*,*,#7453,.T.) ;
#9870=ORIENTED_EDGE('',*,*,#7454,.T.) ;
#9871=ORIENTED_EDGE('',*,*,#7455,.T.) ;
#9872=ORIENTED_EDGE('',*,*,#7456,.T.) ;
#9873=ORIENTED_EDGE('',*,*,#7457,.T.) ;
#9874=ORIENTED_EDGE('',*,*,#7458,.T.) ;
#9875=ORIENTED_EDGE('',*,*,#7459,.T.) ;
#9876=ORIENTED_EDGE('',*,*,#7460,.T.) ;
#9877=ORIENTED_EDGE('',*,*,#7461,.T.) ;
#9878=ORIENTED_EDGE('',*,*,#7462,.T.) ;
#9879=ORIENTED_EDGE('',*,*,#7463,.T.) ;
#9880=ORIENTED_EDGE('',*,*,#7464,.T.) ;
#9881=ORIENTED_EDGE('',*,*,#7465,.T.) ;
#9882=ORIENTED_EDGE('',*,*,#7466,.T.) ;
#9883=ORIENTED_EDGE('',*,*,#7467,.T.) ;
#9884=ORIENTED_EDGE('',*,*,#7467,.F.) ;
#9885=ORIENTED_EDGE('',*,*,#7468,.T.) ;
#9886=ORIENTED_EDGE('',*,*,#7469,.T.) ;
#9887=ORIENTED_EDGE('',*,*,#7470,.T.) ;
#9888=ORIENTED_EDGE('',*,*,#7471,.T.) ;
#9889=ORIENTED_EDGE('',*,*,#7472,.T.) ;
#9890=ORIENTED_EDGE('',*,*,#7473,.T.) ;
#9891=ORIENTED_EDGE('',*,*,#7474,.T.) ;
#9892=ORIENTED_EDGE('',*,*,#7475,.T.) ;
#9893=ORIENTED_EDGE('',*,*,#7476,.T.) ;
#9894=ORIENTED_EDGE('',*,*,#7477,.T.) ;
#9895=ORIENTED_EDGE('',*,*,#7478,.T.) ;
#9896=ORIENTED_EDGE('',*,*,#7479,.F.) ;
#9897=ORIENTED_EDGE('',*,*,#7479,.T.) ;
#9898=ORIENTED_EDGE('',*,*,#7480,.T.) ;
#9899=ORIENTED_EDGE('',*,*,#7481,.T.) ;
#9900=ORIENTED_EDGE('',*,*,#7482,.T.) ;
#9901=ORIENTED_EDGE('',*,*,#7483,.T.) ;
#9902=ORIENTED_EDGE('',*,*,#7484,.T.) ;
#9903=ORIENTED_EDGE('',*,*,#7485,.T.) ;
#9904=ORIENTED_EDGE('',*,*,#7486,.T.) ;
#9905=ORIENTED_EDGE('',*,*,#7487,.T.) ;
#9906=ORIENTED_EDGE('',*,*,#7488,.T.) ;
#9907=ORIENTED_EDGE('',*,*,#7489,.T.) ;
#9908=ORIENTED_EDGE('',*,*,#7490,.T.) ;
#9909=ORIENTED_EDGE('',*,*,#7491,.T.) ;
#9910=ORIENTED_EDGE('',*,*,#7492,.T.) ;
#9911=ORIENTED_EDGE('',*,*,#7493,.T.) ;
#9912=ORIENTED_EDGE('',*,*,#7494,.T.) ;
#9913=ORIENTED_EDGE('',*,*,#7495,.T.) ;
#9914=ORIENTED_EDGE('',*,*,#7495,.F.) ;
#9915=ORIENTED_EDGE('',*,*,#7496,.T.) ;
#9916=ORIENTED_EDGE('',*,*,#7497,.T.) ;
#9917=ORIENTED_EDGE('',*,*,#7498,.T.) ;
#9918=ORIENTED_EDGE('',*,*,#7499,.T.) ;
#9919=ORIENTED_EDGE('',*,*,#7500,.F.) ;
#9920=ORIENTED_EDGE('',*,*,#7501,.T.) ;
#9921=ORIENTED_EDGE('',*,*,#7502,.F.) ;
#9922=ORIENTED_EDGE('',*,*,#7503,.F.) ;
#9923=ORIENTED_EDGE('',*,*,#7390,.F.) ;
#9924=ORIENTED_EDGE('',*,*,#7504,.F.) ;
#9925=ORIENTED_EDGE('',*,*,#7501,.F.) ;
#9926=ORIENTED_EDGE('',*,*,#7500,.T.) ;
#9927=ORIENTED_EDGE('',*,*,#7503,.T.) ;
#9928=ORIENTED_EDGE('',*,*,#7505,.T.) ;
#9929=ORIENTED_EDGE('',*,*,#7506,.F.) ;
#9930=ORIENTED_EDGE('',*,*,#7392,.F.) ;
#9931=ORIENTED_EDGE('',*,*,#7507,.F.) ;
#9932=ORIENTED_EDGE('',*,*,#7505,.F.) ;
#9933=ORIENTED_EDGE('',*,*,#7502,.T.) ;
#9934=ORIENTED_EDGE('',*,*,#7504,.T.) ;
#9935=ORIENTED_EDGE('',*,*,#7391,.F.) ;
#9936=ORIENTED_EDGE('',*,*,#7506,.T.) ;
#9937=ORIENTED_EDGE('',*,*,#7507,.T.) ;
#9938=ORIENTED_EDGE('',*,*,#7396,.F.) ;
#9939=ORIENTED_EDGE('',*,*,#7394,.F.) ;
#9940=ORIENTED_EDGE('',*,*,#7508,.T.) ;
#9941=ORIENTED_EDGE('',*,*,#7397,.F.) ;
#9942=ORIENTED_EDGE('',*,*,#7509,.F.) ;
#9943=ORIENTED_EDGE('',*,*,#7398,.F.) ;
#9944=ORIENTED_EDGE('',*,*,#7508,.F.) ;
#9945=ORIENTED_EDGE('',*,*,#7393,.F.) ;
#9946=ORIENTED_EDGE('',*,*,#7509,.T.) ;
#9947=ORIENTED_EDGE('',*,*,#7400,.F.) ;
#9948=ORIENTED_EDGE('',*,*,#7510,.T.) ;
#9949=ORIENTED_EDGE('',*,*,#7401,.F.) ;
#9950=ORIENTED_EDGE('',*,*,#7511,.F.) ;
#9951=ORIENTED_EDGE('',*,*,#7402,.F.) ;
#9952=ORIENTED_EDGE('',*,*,#7510,.F.) ;
#9953=ORIENTED_EDGE('',*,*,#7399,.F.) ;
#9954=ORIENTED_EDGE('',*,*,#7511,.T.) ;
#9955=ORIENTED_EDGE('',*,*,#7404,.F.) ;
#9956=ORIENTED_EDGE('',*,*,#7512,.T.) ;
#9957=ORIENTED_EDGE('',*,*,#7405,.F.) ;
#9958=ORIENTED_EDGE('',*,*,#7513,.F.) ;
#9959=ORIENTED_EDGE('',*,*,#7406,.F.) ;
#9960=ORIENTED_EDGE('',*,*,#7512,.F.) ;
#9961=ORIENTED_EDGE('',*,*,#7403,.F.) ;
#9962=ORIENTED_EDGE('',*,*,#7513,.T.) ;
#9963=ORIENTED_EDGE('',*,*,#7408,.F.) ;
#9964=ORIENTED_EDGE('',*,*,#7514,.T.) ;
#9965=ORIENTED_EDGE('',*,*,#7409,.F.) ;
#9966=ORIENTED_EDGE('',*,*,#7515,.F.) ;
#9967=ORIENTED_EDGE('',*,*,#7516,.F.) ;
#9968=ORIENTED_EDGE('',*,*,#7412,.F.) ;
#9969=ORIENTED_EDGE('',*,*,#7410,.F.) ;
#9970=ORIENTED_EDGE('',*,*,#7514,.F.) ;
#9971=ORIENTED_EDGE('',*,*,#7407,.F.) ;
#9972=ORIENTED_EDGE('',*,*,#7516,.T.) ;
#9973=ORIENTED_EDGE('',*,*,#7517,.T.) ;
#9974=ORIENTED_EDGE('',*,*,#7518,.F.) ;
#9975=ORIENTED_EDGE('',*,*,#7519,.F.) ;
#9976=ORIENTED_EDGE('',*,*,#7414,.F.) ;
#9977=ORIENTED_EDGE('',*,*,#7520,.F.) ;
#9978=ORIENTED_EDGE('',*,*,#7517,.F.) ;
#9979=ORIENTED_EDGE('',*,*,#7515,.T.) ;
#9980=ORIENTED_EDGE('',*,*,#7413,.F.) ;
#9981=ORIENTED_EDGE('',*,*,#7519,.T.) ;
#9982=ORIENTED_EDGE('',*,*,#7521,.T.) ;
#9983=ORIENTED_EDGE('',*,*,#7522,.F.) ;
#9984=ORIENTED_EDGE('',*,*,#7416,.F.) ;
#9985=ORIENTED_EDGE('',*,*,#7523,.F.) ;
#9986=ORIENTED_EDGE('',*,*,#7521,.F.) ;
#9987=ORIENTED_EDGE('',*,*,#7518,.T.) ;
#9988=ORIENTED_EDGE('',*,*,#7520,.T.) ;
#9989=ORIENTED_EDGE('',*,*,#7415,.F.) ;
#9990=ORIENTED_EDGE('',*,*,#7522,.T.) ;
#9991=ORIENTED_EDGE('',*,*,#7524,.T.) ;
#9992=ORIENTED_EDGE('',*,*,#7525,.F.) ;
#9993=ORIENTED_EDGE('',*,*,#7526,.F.) ;
#9994=ORIENTED_EDGE('',*,*,#7418,.F.) ;
#9995=ORIENTED_EDGE('',*,*,#7527,.F.) ;
#9996=ORIENTED_EDGE('',*,*,#7524,.F.) ;
#9997=ORIENTED_EDGE('',*,*,#7523,.T.) ;
#9998=ORIENTED_EDGE('',*,*,#7417,.F.) ;
#9999=ORIENTED_EDGE('',*,*,#7526,.T.) ;
#10000=ORIENTED_EDGE('',*,*,#7528,.T.) ;
#10001=ORIENTED_EDGE('',*,*,#7529,.F.) ;
#10002=ORIENTED_EDGE('',*,*,#7420,.F.) ;
#10003=ORIENTED_EDGE('',*,*,#7530,.F.) ;
#10004=ORIENTED_EDGE('',*,*,#7528,.F.) ;
#10005=ORIENTED_EDGE('',*,*,#7525,.T.) ;
#10006=ORIENTED_EDGE('',*,*,#7527,.T.) ;
#10007=ORIENTED_EDGE('',*,*,#7419,.F.) ;
#10008=ORIENTED_EDGE('',*,*,#7529,.T.) ;
#10009=ORIENTED_EDGE('',*,*,#7530,.T.) ;
#10010=ORIENTED_EDGE('',*,*,#7424,.F.) ;
#10011=ORIENTED_EDGE('',*,*,#7422,.F.) ;
#10012=ORIENTED_EDGE('',*,*,#7531,.T.) ;
#10013=ORIENTED_EDGE('',*,*,#7425,.F.) ;
#10014=ORIENTED_EDGE('',*,*,#7532,.F.) ;
#10015=ORIENTED_EDGE('',*,*,#7426,.F.) ;
#10016=ORIENTED_EDGE('',*,*,#7531,.F.) ;
#10017=ORIENTED_EDGE('',*,*,#7421,.F.) ;
#10018=ORIENTED_EDGE('',*,*,#7532,.T.) ;
#10019=ORIENTED_EDGE('',*,*,#7428,.F.) ;
#10020=ORIENTED_EDGE('',*,*,#7533,.T.) ;
#10021=ORIENTED_EDGE('',*,*,#7429,.F.) ;
#10022=ORIENTED_EDGE('',*,*,#7534,.F.) ;
#10023=ORIENTED_EDGE('',*,*,#7430,.F.) ;
#10024=ORIENTED_EDGE('',*,*,#7533,.F.) ;
#10025=ORIENTED_EDGE('',*,*,#7427,.F.) ;
#10026=ORIENTED_EDGE('',*,*,#7534,.T.) ;
#10027=ORIENTED_EDGE('',*,*,#7432,.F.) ;
#10028=ORIENTED_EDGE('',*,*,#7535,.T.) ;
#10029=ORIENTED_EDGE('',*,*,#7433,.F.) ;
#10030=ORIENTED_EDGE('',*,*,#7536,.F.) ;
#10031=ORIENTED_EDGE('',*,*,#7434,.F.) ;
#10032=ORIENTED_EDGE('',*,*,#7535,.F.) ;
#10033=ORIENTED_EDGE('',*,*,#7431,.F.) ;
#10034=ORIENTED_EDGE('',*,*,#7536,.T.) ;
#10035=ORIENTED_EDGE('',*,*,#7436,.F.) ;
#10036=ORIENTED_EDGE('',*,*,#7537,.T.) ;
#10037=ORIENTED_EDGE('',*,*,#7437,.F.) ;
#10038=ORIENTED_EDGE('',*,*,#7538,.F.) ;
#10039=ORIENTED_EDGE('',*,*,#7539,.F.) ;
#10040=ORIENTED_EDGE('',*,*,#7440,.F.) ;
#10041=ORIENTED_EDGE('',*,*,#7438,.F.) ;
#10042=ORIENTED_EDGE('',*,*,#7537,.F.) ;
#10043=ORIENTED_EDGE('',*,*,#7435,.F.) ;
#10044=ORIENTED_EDGE('',*,*,#7539,.T.) ;
#10045=ORIENTED_EDGE('',*,*,#7540,.T.) ;
#10046=ORIENTED_EDGE('',*,*,#7541,.F.) ;
#10047=ORIENTED_EDGE('',*,*,#7542,.F.) ;
#10048=ORIENTED_EDGE('',*,*,#7442,.F.) ;
#10049=ORIENTED_EDGE('',*,*,#7543,.F.) ;
#10050=ORIENTED_EDGE('',*,*,#7540,.F.) ;
#10051=ORIENTED_EDGE('',*,*,#7538,.T.) ;
#10052=ORIENTED_EDGE('',*,*,#7441,.F.) ;
#10053=ORIENTED_EDGE('',*,*,#7542,.T.) ;
#10054=ORIENTED_EDGE('',*,*,#7544,.T.) ;
#10055=ORIENTED_EDGE('',*,*,#7545,.F.) ;
#10056=ORIENTED_EDGE('',*,*,#7444,.F.) ;
#10057=ORIENTED_EDGE('',*,*,#7546,.F.) ;
#10058=ORIENTED_EDGE('',*,*,#7544,.F.) ;
#10059=ORIENTED_EDGE('',*,*,#7541,.T.) ;
#10060=ORIENTED_EDGE('',*,*,#7543,.T.) ;
#10061=ORIENTED_EDGE('',*,*,#7443,.F.) ;
#10062=ORIENTED_EDGE('',*,*,#7545,.T.) ;
#10063=ORIENTED_EDGE('',*,*,#7547,.T.) ;
#10064=ORIENTED_EDGE('',*,*,#7548,.F.) ;
#10065=ORIENTED_EDGE('',*,*,#7549,.F.) ;
#10066=ORIENTED_EDGE('',*,*,#7446,.F.) ;
#10067=ORIENTED_EDGE('',*,*,#7550,.F.) ;
#10068=ORIENTED_EDGE('',*,*,#7547,.F.) ;
#10069=ORIENTED_EDGE('',*,*,#7546,.T.) ;
#10070=ORIENTED_EDGE('',*,*,#7445,.F.) ;
#10071=ORIENTED_EDGE('',*,*,#7549,.T.) ;
#10072=ORIENTED_EDGE('',*,*,#7551,.T.) ;
#10073=ORIENTED_EDGE('',*,*,#7552,.F.) ;
#10074=ORIENTED_EDGE('',*,*,#7448,.F.) ;
#10075=ORIENTED_EDGE('',*,*,#7553,.F.) ;
#10076=ORIENTED_EDGE('',*,*,#7551,.F.) ;
#10077=ORIENTED_EDGE('',*,*,#7548,.T.) ;
#10078=ORIENTED_EDGE('',*,*,#7550,.T.) ;
#10079=ORIENTED_EDGE('',*,*,#7447,.F.) ;
#10080=ORIENTED_EDGE('',*,*,#7552,.T.) ;
#10081=ORIENTED_EDGE('',*,*,#7553,.T.) ;
#10082=ORIENTED_EDGE('',*,*,#7452,.F.) ;
#10083=ORIENTED_EDGE('',*,*,#7450,.F.) ;
#10084=ORIENTED_EDGE('',*,*,#7554,.T.) ;
#10085=ORIENTED_EDGE('',*,*,#7453,.F.) ;
#10086=ORIENTED_EDGE('',*,*,#7555,.F.) ;
#10087=ORIENTED_EDGE('',*,*,#7454,.F.) ;
#10088=ORIENTED_EDGE('',*,*,#7554,.F.) ;
#10089=ORIENTED_EDGE('',*,*,#7449,.F.) ;
#10090=ORIENTED_EDGE('',*,*,#7555,.T.) ;
#10091=ORIENTED_EDGE('',*,*,#7456,.F.) ;
#10092=ORIENTED_EDGE('',*,*,#7556,.T.) ;
#10093=ORIENTED_EDGE('',*,*,#7457,.F.) ;
#10094=ORIENTED_EDGE('',*,*,#7557,.F.) ;
#10095=ORIENTED_EDGE('',*,*,#7458,.F.) ;
#10096=ORIENTED_EDGE('',*,*,#7556,.F.) ;
#10097=ORIENTED_EDGE('',*,*,#7455,.F.) ;
#10098=ORIENTED_EDGE('',*,*,#7557,.T.) ;
#10099=ORIENTED_EDGE('',*,*,#7460,.F.) ;
#10100=ORIENTED_EDGE('',*,*,#7558,.T.) ;
#10101=ORIENTED_EDGE('',*,*,#7461,.F.) ;
#10102=ORIENTED_EDGE('',*,*,#7559,.F.) ;
#10103=ORIENTED_EDGE('',*,*,#7462,.F.) ;
#10104=ORIENTED_EDGE('',*,*,#7558,.F.) ;
#10105=ORIENTED_EDGE('',*,*,#7459,.F.) ;
#10106=ORIENTED_EDGE('',*,*,#7559,.T.) ;
#10107=ORIENTED_EDGE('',*,*,#7464,.F.) ;
#10108=ORIENTED_EDGE('',*,*,#7560,.T.) ;
#10109=ORIENTED_EDGE('',*,*,#7465,.F.) ;
#10110=ORIENTED_EDGE('',*,*,#7561,.F.) ;
#10111=ORIENTED_EDGE('',*,*,#7562,.F.) ;
#10112=ORIENTED_EDGE('',*,*,#7468,.F.) ;
#10113=ORIENTED_EDGE('',*,*,#7466,.F.) ;
#10114=ORIENTED_EDGE('',*,*,#7560,.F.) ;
#10115=ORIENTED_EDGE('',*,*,#7463,.F.) ;
#10116=ORIENTED_EDGE('',*,*,#7562,.T.) ;
#10117=ORIENTED_EDGE('',*,*,#7563,.T.) ;
#10118=ORIENTED_EDGE('',*,*,#7564,.F.) ;
#10119=ORIENTED_EDGE('',*,*,#7565,.F.) ;
#10120=ORIENTED_EDGE('',*,*,#7470,.F.) ;
#10121=ORIENTED_EDGE('',*,*,#7566,.F.) ;
#10122=ORIENTED_EDGE('',*,*,#7563,.F.) ;
#10123=ORIENTED_EDGE('',*,*,#7561,.T.) ;
#10124=ORIENTED_EDGE('',*,*,#7469,.F.) ;
#10125=ORIENTED_EDGE('',*,*,#7565,.T.) ;
#10126=ORIENTED_EDGE('',*,*,#7567,.T.) ;
#10127=ORIENTED_EDGE('',*,*,#7568,.F.) ;
#10128=ORIENTED_EDGE('',*,*,#7472,.F.) ;
#10129=ORIENTED_EDGE('',*,*,#7569,.F.) ;
#10130=ORIENTED_EDGE('',*,*,#7567,.F.) ;
#10131=ORIENTED_EDGE('',*,*,#7564,.T.) ;
#10132=ORIENTED_EDGE('',*,*,#7566,.T.) ;
#10133=ORIENTED_EDGE('',*,*,#7471,.F.) ;
#10134=ORIENTED_EDGE('',*,*,#7568,.T.) ;
#10135=ORIENTED_EDGE('',*,*,#7570,.T.) ;
#10136=ORIENTED_EDGE('',*,*,#7571,.F.) ;
#10137=ORIENTED_EDGE('',*,*,#7572,.F.) ;
#10138=ORIENTED_EDGE('',*,*,#7474,.F.) ;
#10139=ORIENTED_EDGE('',*,*,#7573,.F.) ;
#10140=ORIENTED_EDGE('',*,*,#7570,.F.) ;
#10141=ORIENTED_EDGE('',*,*,#7569,.T.) ;
#10142=ORIENTED_EDGE('',*,*,#7473,.F.) ;
#10143=ORIENTED_EDGE('',*,*,#7572,.T.) ;
#10144=ORIENTED_EDGE('',*,*,#7574,.T.) ;
#10145=ORIENTED_EDGE('',*,*,#7575,.F.) ;
#10146=ORIENTED_EDGE('',*,*,#7476,.F.) ;
#10147=ORIENTED_EDGE('',*,*,#7576,.F.) ;
#10148=ORIENTED_EDGE('',*,*,#7574,.F.) ;
#10149=ORIENTED_EDGE('',*,*,#7571,.T.) ;
#10150=ORIENTED_EDGE('',*,*,#7573,.T.) ;
#10151=ORIENTED_EDGE('',*,*,#7475,.F.) ;
#10152=ORIENTED_EDGE('',*,*,#7575,.T.) ;
#10153=ORIENTED_EDGE('',*,*,#7576,.T.) ;
#10154=ORIENTED_EDGE('',*,*,#7480,.F.) ;
#10155=ORIENTED_EDGE('',*,*,#7478,.F.) ;
#10156=ORIENTED_EDGE('',*,*,#7577,.T.) ;
#10157=ORIENTED_EDGE('',*,*,#7481,.F.) ;
#10158=ORIENTED_EDGE('',*,*,#7578,.F.) ;
#10159=ORIENTED_EDGE('',*,*,#7482,.F.) ;
#10160=ORIENTED_EDGE('',*,*,#7577,.F.) ;
#10161=ORIENTED_EDGE('',*,*,#7477,.F.) ;
#10162=ORIENTED_EDGE('',*,*,#7578,.T.) ;
#10163=ORIENTED_EDGE('',*,*,#7484,.F.) ;
#10164=ORIENTED_EDGE('',*,*,#7579,.T.) ;
#10165=ORIENTED_EDGE('',*,*,#7485,.F.) ;
#10166=ORIENTED_EDGE('',*,*,#7580,.F.) ;
#10167=ORIENTED_EDGE('',*,*,#7486,.F.) ;
#10168=ORIENTED_EDGE('',*,*,#7579,.F.) ;
#10169=ORIENTED_EDGE('',*,*,#7483,.F.) ;
#10170=ORIENTED_EDGE('',*,*,#7580,.T.) ;
#10171=ORIENTED_EDGE('',*,*,#7488,.F.) ;
#10172=ORIENTED_EDGE('',*,*,#7581,.T.) ;
#10173=ORIENTED_EDGE('',*,*,#7489,.F.) ;
#10174=ORIENTED_EDGE('',*,*,#7582,.F.) ;
#10175=ORIENTED_EDGE('',*,*,#7490,.F.) ;
#10176=ORIENTED_EDGE('',*,*,#7581,.F.) ;
#10177=ORIENTED_EDGE('',*,*,#7487,.F.) ;
#10178=ORIENTED_EDGE('',*,*,#7582,.T.) ;
#10179=ORIENTED_EDGE('',*,*,#7492,.F.) ;
#10180=ORIENTED_EDGE('',*,*,#7583,.T.) ;
#10181=ORIENTED_EDGE('',*,*,#7493,.F.) ;
#10182=ORIENTED_EDGE('',*,*,#7584,.F.) ;
#10183=ORIENTED_EDGE('',*,*,#7585,.F.) ;
#10184=ORIENTED_EDGE('',*,*,#7496,.F.) ;
#10185=ORIENTED_EDGE('',*,*,#7494,.F.) ;
#10186=ORIENTED_EDGE('',*,*,#7583,.F.) ;
#10187=ORIENTED_EDGE('',*,*,#7491,.F.) ;
#10188=ORIENTED_EDGE('',*,*,#7585,.T.) ;
#10189=ORIENTED_EDGE('',*,*,#7586,.T.) ;
#10190=ORIENTED_EDGE('',*,*,#7587,.F.) ;
#10191=ORIENTED_EDGE('',*,*,#7588,.F.) ;
#10192=ORIENTED_EDGE('',*,*,#7498,.F.) ;
#10193=ORIENTED_EDGE('',*,*,#7589,.F.) ;
#10194=ORIENTED_EDGE('',*,*,#7586,.F.) ;
#10195=ORIENTED_EDGE('',*,*,#7584,.T.) ;
#10196=ORIENTED_EDGE('',*,*,#7497,.F.) ;
#10197=ORIENTED_EDGE('',*,*,#7588,.T.) ;
#10198=ORIENTED_EDGE('',*,*,#7590,.T.) ;
#10199=ORIENTED_EDGE('',*,*,#7591,.F.) ;
#10200=ORIENTED_EDGE('',*,*,#7590,.F.) ;
#10201=ORIENTED_EDGE('',*,*,#7587,.T.) ;
#10202=ORIENTED_EDGE('',*,*,#7589,.T.) ;
#10203=ORIENTED_EDGE('',*,*,#7499,.F.) ;
#10204=ORIENTED_EDGE('',*,*,#7591,.T.) ;
#12148=PLANE('',#14406) ;
#12149=PLANE('',#14494) ;
#12639=ADVANCED_FACE('',(#3244),#359,.T.) ;
#12640=ADVANCED_FACE('',(#3245),#360,.T.) ;
#12641=ADVANCED_FACE('',(#3246),#361,.T.) ;
#12642=ADVANCED_FACE('',(#3247),#362,.T.) ;
#12643=ADVANCED_FACE('',(#3248),#363,.T.) ;
#12644=ADVANCED_FACE('',(#3249),#364,.T.) ;
#12645=ADVANCED_FACE('',(#3250),#365,.T.) ;
#12646=ADVANCED_FACE('',(#3251),#366,.T.) ;
#12647=ADVANCED_FACE('',(#3252),#367,.T.) ;
#12648=ADVANCED_FACE('',(#3253),#368,.T.) ;
#12649=ADVANCED_FACE('',(#3254),#369,.T.) ;
#12650=ADVANCED_FACE('',(#3255),#370,.T.) ;
#12651=ADVANCED_FACE('',(#3256),#371,.T.) ;
#12652=ADVANCED_FACE('',(#3257),#372,.T.) ;
#12653=ADVANCED_FACE('',(#3258),#373,.T.) ;
#12654=ADVANCED_FACE('',(#3259),#374,.T.) ;
#12655=ADVANCED_FACE('',(#3260),#375,.T.) ;
#12656=ADVANCED_FACE('',(#3261),#376,.T.) ;
#12657=ADVANCED_FACE('',(#3262),#377,.T.) ;
#12658=ADVANCED_FACE('',(#3263),#378,.T.) ;
#12659=ADVANCED_FACE('',(#3264),#379,.T.) ;
#12660=ADVANCED_FACE('',(#3265),#380,.T.) ;
#12661=ADVANCED_FACE('',(#3266),#381,.T.) ;
#12662=ADVANCED_FACE('',(#3267),#382,.T.) ;
#12663=ADVANCED_FACE('',(#3268),#383,.T.) ;
#12664=ADVANCED_FACE('',(#3269),#384,.T.) ;
#12665=ADVANCED_FACE('',(#3270),#385,.T.) ;
#12666=ADVANCED_FACE('',(#3271),#386,.T.) ;
#12667=ADVANCED_FACE('',(#3272),#387,.T.) ;
#12668=ADVANCED_FACE('',(#3273),#388,.T.) ;
#12669=ADVANCED_FACE('',(#3274),#389,.T.) ;
#12670=ADVANCED_FACE('',(#3275),#2812,.T.) ;
#12671=ADVANCED_FACE('',(#3276),#12148,.T.) ;
#12672=ADVANCED_FACE('',(#3277),#2813,.T.) ;
#12673=ADVANCED_FACE('',(#3278),#2814,.T.) ;
#12674=ADVANCED_FACE('',(#3279),#2815,.T.) ;
#12675=ADVANCED_FACE('',(#3280),#2816,.T.) ;
#12676=ADVANCED_FACE('',(#3281),#2817,.T.) ;
#12677=ADVANCED_FACE('',(#3282),#2818,.T.) ;
#12678=ADVANCED_FACE('',(#3283),#2819,.T.) ;
#12679=ADVANCED_FACE('',(#3284),#2820,.T.) ;
#12680=ADVANCED_FACE('',(#3285),#2821,.T.) ;
#12681=ADVANCED_FACE('',(#3286),#2822,.T.) ;
#12682=ADVANCED_FACE('',(#3287),#2823,.T.) ;
#12683=ADVANCED_FACE('',(#3288),#2824,.T.) ;
#12684=ADVANCED_FACE('',(#3289),#2825,.T.) ;
#12685=ADVANCED_FACE('',(#3290),#2826,.T.) ;
#12686=ADVANCED_FACE('',(#3291),#2827,.T.) ;
#12687=ADVANCED_FACE('',(#3292),#2828,.T.) ;
#12688=ADVANCED_FACE('',(#3293),#2829,.T.) ;
#12689=ADVANCED_FACE('',(#3294),#2830,.T.) ;
#12690=ADVANCED_FACE('',(#3295),#2831,.T.) ;
#12691=ADVANCED_FACE('',(#3296),#2832,.T.) ;
#12692=ADVANCED_FACE('',(#3297),#2833,.T.) ;
#12693=ADVANCED_FACE('',(#3298),#2834,.T.) ;
#12694=ADVANCED_FACE('',(#3299),#2835,.T.) ;
#12695=ADVANCED_FACE('',(#3300),#2836,.T.) ;
#12696=ADVANCED_FACE('',(#3301),#2837,.T.) ;
#12697=ADVANCED_FACE('',(#3302),#2838,.T.) ;
#12698=ADVANCED_FACE('',(#3303),#2839,.T.) ;
#12699=ADVANCED_FACE('',(#3304),#2840,.T.) ;
#12700=ADVANCED_FACE('',(#3305),#2841,.T.) ;
#12701=ADVANCED_FACE('',(#3306),#2842,.T.) ;
#12702=ADVANCED_FACE('',(#3307),#2843,.T.) ;
#12703=ADVANCED_FACE('',(#3308),#12149,.T.) ;
#13132=CLOSED_SHELL('',(#12639,#12640,#12641,#12642,#12643,#12644,#12645,
#12646,#12647,#12648,#12649,#12650,#12651,#12652,#12653,#12654,#12655,#12656,
#12657,#12658,#12659,#12660,#12661,#12662,#12663,#12664,#12665,#12666,#12667,
#12668,#12669,#12670,#12671,#12672,#12673,#12674,#12675,#12676,#12677,#12678,
#12679,#12680,#12681,#12682,#12683,#12684,#12685,#12686,#12687,#12688,#12689,
#12690,#12691,#12692,#12693,#12694,#12695,#12696,#12697,#12698,#12699,#12700,
#12701,#12702,#12703)) ;
#14259=AXIS2_PLACEMENT_3D('',#21209,#16959,#16960) ;
#14260=AXIS2_PLACEMENT_3D('',#21210,#16961,#16962) ;
#14261=AXIS2_PLACEMENT_3D('',#21213,#16963,#16964) ;
#14262=AXIS2_PLACEMENT_3D('',#21214,#16965,#16966) ;
#14263=AXIS2_PLACEMENT_3D('',#21215,#16967,#16968) ;
#14264=AXIS2_PLACEMENT_3D('',#21218,#16969,#16970) ;
#14265=AXIS2_PLACEMENT_3D('',#21220,#16971,#16972) ;
#14266=AXIS2_PLACEMENT_3D('',#21222,#16973,#16974) ;
#14267=AXIS2_PLACEMENT_3D('',#21224,#16975,#16976) ;
#14268=AXIS2_PLACEMENT_3D('',#21225,#16977,#16978) ;
#14269=AXIS2_PLACEMENT_3D('',#21226,#16979,#16980) ;
#14270=AXIS2_PLACEMENT_3D('',#21229,#16981,#16982) ;
#14271=AXIS2_PLACEMENT_3D('',#21231,#16983,#16984) ;
#14272=AXIS2_PLACEMENT_3D('',#21233,#16985,#16986) ;
#14273=AXIS2_PLACEMENT_3D('',#21234,#16987,#16988) ;
#14274=AXIS2_PLACEMENT_3D('',#21235,#16989,#16990) ;
#14275=AXIS2_PLACEMENT_3D('',#21238,#16991,#16992) ;
#14276=AXIS2_PLACEMENT_3D('',#21240,#16993,#16994) ;
#14277=AXIS2_PLACEMENT_3D('',#21242,#16995,#16996) ;
#14278=AXIS2_PLACEMENT_3D('',#21243,#16997,#16998) ;
#14279=AXIS2_PLACEMENT_3D('',#21244,#16999,#17000) ;
#14280=AXIS2_PLACEMENT_3D('',#21247,#17001,#17002) ;
#14281=AXIS2_PLACEMENT_3D('',#21249,#17003,#17004) ;
#14282=AXIS2_PLACEMENT_3D('',#21251,#17005,#17006) ;
#14283=AXIS2_PLACEMENT_3D('',#21252,#17007,#17008) ;
#14284=AXIS2_PLACEMENT_3D('',#21253,#17009,#17010) ;
#14285=AXIS2_PLACEMENT_3D('',#21256,#17011,#17012) ;
#14286=AXIS2_PLACEMENT_3D('',#21258,#17013,#17014) ;
#14287=AXIS2_PLACEMENT_3D('',#21260,#17015,#17016) ;
#14288=AXIS2_PLACEMENT_3D('',#21262,#17017,#17018) ;
#14289=AXIS2_PLACEMENT_3D('',#21263,#17019,#17020) ;
#14290=AXIS2_PLACEMENT_3D('',#21264,#17021,#17022) ;
#14291=AXIS2_PLACEMENT_3D('',#21267,#17023,#17024) ;
#14292=AXIS2_PLACEMENT_3D('',#21268,#17025,#17026) ;
#14293=AXIS2_PLACEMENT_3D('',#21269,#17027,#17028) ;
#14294=AXIS2_PLACEMENT_3D('',#21272,#17029,#17030) ;
#14295=AXIS2_PLACEMENT_3D('',#21273,#17031,#17032) ;
#14296=AXIS2_PLACEMENT_3D('',#21274,#17033,#17034) ;
#14297=AXIS2_PLACEMENT_3D('',#21277,#17035,#17036) ;
#14298=AXIS2_PLACEMENT_3D('',#21278,#17037,#17038) ;
#14299=AXIS2_PLACEMENT_3D('',#21279,#17039,#17040) ;
#14300=AXIS2_PLACEMENT_3D('',#21282,#17041,#17042) ;
#14301=AXIS2_PLACEMENT_3D('',#21284,#17043,#17044) ;
#14302=AXIS2_PLACEMENT_3D('',#21286,#17045,#17046) ;
#14303=AXIS2_PLACEMENT_3D('',#21288,#17047,#17048) ;
#14304=AXIS2_PLACEMENT_3D('',#21289,#17049,#17050) ;
#14305=AXIS2_PLACEMENT_3D('',#21290,#17051,#17052) ;
#14306=AXIS2_PLACEMENT_3D('',#21293,#17053,#17054) ;
#14307=AXIS2_PLACEMENT_3D('',#21295,#17055,#17056) ;
#14308=AXIS2_PLACEMENT_3D('',#21297,#17057,#17058) ;
#14309=AXIS2_PLACEMENT_3D('',#21298,#17059,#17060) ;
#14310=AXIS2_PLACEMENT_3D('',#21299,#17061,#17062) ;
#14311=AXIS2_PLACEMENT_3D('',#21302,#17063,#17064) ;
#14312=AXIS2_PLACEMENT_3D('',#21304,#17065,#17066) ;
#14313=AXIS2_PLACEMENT_3D('',#21306,#17067,#17068) ;
#14314=AXIS2_PLACEMENT_3D('',#21307,#17069,#17070) ;
#14315=AXIS2_PLACEMENT_3D('',#21308,#17071,#17072) ;
#14316=AXIS2_PLACEMENT_3D('',#21311,#17073,#17074) ;
#14317=AXIS2_PLACEMENT_3D('',#21313,#17075,#17076) ;
#14318=AXIS2_PLACEMENT_3D('',#21315,#17077,#17078) ;
#14319=AXIS2_PLACEMENT_3D('',#21316,#17079,#17080) ;
#14320=AXIS2_PLACEMENT_3D('',#21317,#17081,#17082) ;
#14321=AXIS2_PLACEMENT_3D('',#21320,#17083,#17084) ;
#14322=AXIS2_PLACEMENT_3D('',#21322,#17085,#17086) ;
#14323=AXIS2_PLACEMENT_3D('',#21324,#17087,#17088) ;
#14324=AXIS2_PLACEMENT_3D('',#21326,#17089,#17090) ;
#14325=AXIS2_PLACEMENT_3D('',#21327,#17091,#17092) ;
#14326=AXIS2_PLACEMENT_3D('',#21328,#17093,#17094) ;
#14327=AXIS2_PLACEMENT_3D('',#21331,#17095,#17096) ;
#14328=AXIS2_PLACEMENT_3D('',#21332,#17097,#17098) ;
#14329=AXIS2_PLACEMENT_3D('',#21333,#17099,#17100) ;
#14330=AXIS2_PLACEMENT_3D('',#21336,#17101,#17102) ;
#14331=AXIS2_PLACEMENT_3D('',#21337,#17103,#17104) ;
#14332=AXIS2_PLACEMENT_3D('',#21338,#17105,#17106) ;
#14333=AXIS2_PLACEMENT_3D('',#21341,#17107,#17108) ;
#14334=AXIS2_PLACEMENT_3D('',#21342,#17109,#17110) ;
#14335=AXIS2_PLACEMENT_3D('',#21343,#17111,#17112) ;
#14336=AXIS2_PLACEMENT_3D('',#21346,#17113,#17114) ;
#14337=AXIS2_PLACEMENT_3D('',#21348,#17115,#17116) ;
#14338=AXIS2_PLACEMENT_3D('',#21350,#17117,#17118) ;
#14339=AXIS2_PLACEMENT_3D('',#21352,#17119,#17120) ;
#14340=AXIS2_PLACEMENT_3D('',#21353,#17121,#17122) ;
#14341=AXIS2_PLACEMENT_3D('',#21354,#17123,#17124) ;
#14342=AXIS2_PLACEMENT_3D('',#21357,#17125,#17126) ;
#14343=AXIS2_PLACEMENT_3D('',#21359,#17127,#17128) ;
#14344=AXIS2_PLACEMENT_3D('',#21361,#17129,#17130) ;
#14345=AXIS2_PLACEMENT_3D('',#21362,#17131,#17132) ;
#14346=AXIS2_PLACEMENT_3D('',#21363,#17133,#17134) ;
#14347=AXIS2_PLACEMENT_3D('',#21366,#17135,#17136) ;
#14348=AXIS2_PLACEMENT_3D('',#21368,#17137,#17138) ;
#14349=AXIS2_PLACEMENT_3D('',#21370,#17139,#17140) ;
#14350=AXIS2_PLACEMENT_3D('',#21371,#17141,#17142) ;
#14351=AXIS2_PLACEMENT_3D('',#21372,#17143,#17144) ;
#14352=AXIS2_PLACEMENT_3D('',#21375,#17145,#17146) ;
#14353=AXIS2_PLACEMENT_3D('',#21377,#17147,#17148) ;
#14354=AXIS2_PLACEMENT_3D('',#21379,#17149,#17150) ;
#14355=AXIS2_PLACEMENT_3D('',#21380,#17151,#17152) ;
#14356=AXIS2_PLACEMENT_3D('',#21381,#17153,#17154) ;
#14357=AXIS2_PLACEMENT_3D('',#21384,#17155,#17156) ;
#14358=AXIS2_PLACEMENT_3D('',#21386,#17157,#17158) ;
#14359=AXIS2_PLACEMENT_3D('',#21388,#17159,#17160) ;
#14360=AXIS2_PLACEMENT_3D('',#21390,#17161,#17162) ;
#14361=AXIS2_PLACEMENT_3D('',#21391,#17163,#17164) ;
#14362=AXIS2_PLACEMENT_3D('',#21392,#17165,#17166) ;
#14363=AXIS2_PLACEMENT_3D('',#21395,#17167,#17168) ;
#14364=AXIS2_PLACEMENT_3D('',#21396,#17169,#17170) ;
#14365=AXIS2_PLACEMENT_3D('',#21397,#17171,#17172) ;
#14366=AXIS2_PLACEMENT_3D('',#21400,#17173,#17174) ;
#14367=AXIS2_PLACEMENT_3D('',#21401,#17175,#17176) ;
#14368=AXIS2_PLACEMENT_3D('',#21402,#17177,#17178) ;
#14369=AXIS2_PLACEMENT_3D('',#21405,#17179,#17180) ;
#14370=AXIS2_PLACEMENT_3D('',#21406,#17181,#17182) ;
#14371=AXIS2_PLACEMENT_3D('',#21407,#17183,#17184) ;
#14372=AXIS2_PLACEMENT_3D('',#21410,#17185,#17186) ;
#14373=AXIS2_PLACEMENT_3D('',#21412,#17187,#17188) ;
#14374=AXIS2_PLACEMENT_3D('',#21414,#17189,#17190) ;
#14375=AXIS2_PLACEMENT_3D('',#21416,#17191,#17192) ;
#14376=AXIS2_PLACEMENT_3D('',#21417,#17193,#17194) ;
#14377=AXIS2_PLACEMENT_3D('',#21418,#17195,#17196) ;
#14378=AXIS2_PLACEMENT_3D('',#21421,#17197,#17198) ;
#14379=AXIS2_PLACEMENT_3D('',#21423,#17199,#17200) ;
#14380=AXIS2_PLACEMENT_3D('',#21425,#17201,#17202) ;
#14381=AXIS2_PLACEMENT_3D('',#21426,#17203,#17204) ;
#14382=AXIS2_PLACEMENT_3D('',#21427,#17205,#17206) ;
#14383=AXIS2_PLACEMENT_3D('',#21430,#17207,#17208) ;
#14384=AXIS2_PLACEMENT_3D('',#21432,#17209,#17210) ;
#14385=AXIS2_PLACEMENT_3D('',#21434,#17211,#17212) ;
#14386=AXIS2_PLACEMENT_3D('',#21435,#17213,#17214) ;
#14387=AXIS2_PLACEMENT_3D('',#21436,#17215,#17216) ;
#14388=AXIS2_PLACEMENT_3D('',#21439,#17217,#17218) ;
#14389=AXIS2_PLACEMENT_3D('',#21441,#17219,#17220) ;
#14390=AXIS2_PLACEMENT_3D('',#21443,#17221,#17222) ;
#14391=AXIS2_PLACEMENT_3D('',#21444,#17223,#17224) ;
#14392=AXIS2_PLACEMENT_3D('',#21445,#17225,#17226) ;
#14393=AXIS2_PLACEMENT_3D('',#21448,#17227,#17228) ;
#14394=AXIS2_PLACEMENT_3D('',#21450,#17229,#17230) ;
#14395=AXIS2_PLACEMENT_3D('',#21452,#17231,#17232) ;
#14396=AXIS2_PLACEMENT_3D('',#21454,#17233,#17234) ;
#14397=AXIS2_PLACEMENT_3D('',#21455,#17235,#17236) ;
#14398=AXIS2_PLACEMENT_3D('',#21456,#17237,#17238) ;
#14399=AXIS2_PLACEMENT_3D('',#21459,#17239,#17240) ;
#14400=AXIS2_PLACEMENT_3D('',#21460,#17241,#17242) ;
#14401=AXIS2_PLACEMENT_3D('',#21461,#17243,#17244) ;
#14402=AXIS2_PLACEMENT_3D('',#21463,#17245,#17246) ;
#14403=AXIS2_PLACEMENT_3D('',#21467,#17248,#17249) ;
#14404=AXIS2_PLACEMENT_3D('',#21468,#17250,#17251) ;
#14405=AXIS2_PLACEMENT_3D('',#21469,#17252,#17253) ;
#14406=AXIS2_PLACEMENT_3D('',#21470,#17254,#17255) ;
#14407=AXIS2_PLACEMENT_3D('',#21471,#17256,#17257) ;
#14408=AXIS2_PLACEMENT_3D('',#21474,#17259,#17260) ;
#14409=AXIS2_PLACEMENT_3D('',#21475,#17261,#17262) ;
#14410=AXIS2_PLACEMENT_3D('',#21476,#17263,#17264) ;
#14411=AXIS2_PLACEMENT_3D('',#21478,#17266,#17267) ;
#14412=AXIS2_PLACEMENT_3D('',#21479,#17268,#17269) ;
#14413=AXIS2_PLACEMENT_3D('',#21481,#17271,#17272) ;
#14414=AXIS2_PLACEMENT_3D('',#21482,#17273,#17274) ;
#14415=AXIS2_PLACEMENT_3D('',#21484,#17276,#17277) ;
#14416=AXIS2_PLACEMENT_3D('',#21485,#17278,#17279) ;
#14417=AXIS2_PLACEMENT_3D('',#21488,#17281,#17282) ;
#14418=AXIS2_PLACEMENT_3D('',#21489,#17283,#17284) ;
#14419=AXIS2_PLACEMENT_3D('',#21490,#17285,#17286) ;
#14420=AXIS2_PLACEMENT_3D('',#21494,#17288,#17289) ;
#14421=AXIS2_PLACEMENT_3D('',#21495,#17290,#17291) ;
#14422=AXIS2_PLACEMENT_3D('',#21496,#17292,#17293) ;
#14423=AXIS2_PLACEMENT_3D('',#21497,#17294,#17295) ;
#14424=AXIS2_PLACEMENT_3D('',#21500,#17297,#17298) ;
#14425=AXIS2_PLACEMENT_3D('',#21501,#17299,#17300) ;
#14426=AXIS2_PLACEMENT_3D('',#21502,#17301,#17302) ;
#14427=AXIS2_PLACEMENT_3D('',#21506,#17304,#17305) ;
#14428=AXIS2_PLACEMENT_3D('',#21507,#17306,#17307) ;
#14429=AXIS2_PLACEMENT_3D('',#21508,#17308,#17309) ;
#14430=AXIS2_PLACEMENT_3D('',#21509,#17310,#17311) ;
#14431=AXIS2_PLACEMENT_3D('',#21512,#17313,#17314) ;
#14432=AXIS2_PLACEMENT_3D('',#21513,#17315,#17316) ;
#14433=AXIS2_PLACEMENT_3D('',#21514,#17317,#17318) ;
#14434=AXIS2_PLACEMENT_3D('',#21516,#17320,#17321) ;
#14435=AXIS2_PLACEMENT_3D('',#21517,#17322,#17323) ;
#14436=AXIS2_PLACEMENT_3D('',#21519,#17325,#17326) ;
#14437=AXIS2_PLACEMENT_3D('',#21520,#17327,#17328) ;
#14438=AXIS2_PLACEMENT_3D('',#21522,#17330,#17331) ;
#14439=AXIS2_PLACEMENT_3D('',#21523,#17332,#17333) ;
#14440=AXIS2_PLACEMENT_3D('',#21526,#17335,#17336) ;
#14441=AXIS2_PLACEMENT_3D('',#21527,#17337,#17338) ;
#14442=AXIS2_PLACEMENT_3D('',#21528,#17339,#17340) ;
#14443=AXIS2_PLACEMENT_3D('',#21532,#17342,#17343) ;
#14444=AXIS2_PLACEMENT_3D('',#21533,#17344,#17345) ;
#14445=AXIS2_PLACEMENT_3D('',#21534,#17346,#17347) ;
#14446=AXIS2_PLACEMENT_3D('',#21535,#17348,#17349) ;
#14447=AXIS2_PLACEMENT_3D('',#21538,#17351,#17352) ;
#14448=AXIS2_PLACEMENT_3D('',#21539,#17353,#17354) ;
#14449=AXIS2_PLACEMENT_3D('',#21540,#17355,#17356) ;
#14450=AXIS2_PLACEMENT_3D('',#21544,#17358,#17359) ;
#14451=AXIS2_PLACEMENT_3D('',#21545,#17360,#17361) ;
#14452=AXIS2_PLACEMENT_3D('',#21546,#17362,#17363) ;
#14453=AXIS2_PLACEMENT_3D('',#21547,#17364,#17365) ;
#14454=AXIS2_PLACEMENT_3D('',#21550,#17367,#17368) ;
#14455=AXIS2_PLACEMENT_3D('',#21551,#17369,#17370) ;
#14456=AXIS2_PLACEMENT_3D('',#21552,#17371,#17372) ;
#14457=AXIS2_PLACEMENT_3D('',#21554,#17374,#17375) ;
#14458=AXIS2_PLACEMENT_3D('',#21555,#17376,#17377) ;
#14459=AXIS2_PLACEMENT_3D('',#21557,#17379,#17380) ;
#14460=AXIS2_PLACEMENT_3D('',#21558,#17381,#17382) ;
#14461=AXIS2_PLACEMENT_3D('',#21560,#17384,#17385) ;
#14462=AXIS2_PLACEMENT_3D('',#21561,#17386,#17387) ;
#14463=AXIS2_PLACEMENT_3D('',#21564,#17389,#17390) ;
#14464=AXIS2_PLACEMENT_3D('',#21565,#17391,#17392) ;
#14465=AXIS2_PLACEMENT_3D('',#21566,#17393,#17394) ;
#14466=AXIS2_PLACEMENT_3D('',#21570,#17396,#17397) ;
#14467=AXIS2_PLACEMENT_3D('',#21571,#17398,#17399) ;
#14468=AXIS2_PLACEMENT_3D('',#21572,#17400,#17401) ;
#14469=AXIS2_PLACEMENT_3D('',#21573,#17402,#17403) ;
#14470=AXIS2_PLACEMENT_3D('',#21576,#17405,#17406) ;
#14471=AXIS2_PLACEMENT_3D('',#21577,#17407,#17408) ;
#14472=AXIS2_PLACEMENT_3D('',#21578,#17409,#17410) ;
#14473=AXIS2_PLACEMENT_3D('',#21582,#17412,#17413) ;
#14474=AXIS2_PLACEMENT_3D('',#21583,#17414,#17415) ;
#14475=AXIS2_PLACEMENT_3D('',#21584,#17416,#17417) ;
#14476=AXIS2_PLACEMENT_3D('',#21585,#17418,#17419) ;
#14477=AXIS2_PLACEMENT_3D('',#21588,#17421,#17422) ;
#14478=AXIS2_PLACEMENT_3D('',#21589,#17423,#17424) ;
#14479=AXIS2_PLACEMENT_3D('',#21590,#17425,#17426) ;
#14480=AXIS2_PLACEMENT_3D('',#21592,#17428,#17429) ;
#14481=AXIS2_PLACEMENT_3D('',#21593,#17430,#17431) ;
#14482=AXIS2_PLACEMENT_3D('',#21595,#17433,#17434) ;
#14483=AXIS2_PLACEMENT_3D('',#21596,#17435,#17436) ;
#14484=AXIS2_PLACEMENT_3D('',#21598,#17438,#17439) ;
#14485=AXIS2_PLACEMENT_3D('',#21599,#17440,#17441) ;
#14486=AXIS2_PLACEMENT_3D('',#21602,#17443,#17444) ;
#14487=AXIS2_PLACEMENT_3D('',#21603,#17445,#17446) ;
#14488=AXIS2_PLACEMENT_3D('',#21604,#17447,#17448) ;
#14489=AXIS2_PLACEMENT_3D('',#21608,#17450,#17451) ;
#14490=AXIS2_PLACEMENT_3D('',#21609,#17452,#17453) ;
#14491=AXIS2_PLACEMENT_3D('',#21610,#17454,#17455) ;
#14492=AXIS2_PLACEMENT_3D('',#21611,#17456,#17457) ;
#14493=AXIS2_PLACEMENT_3D('',#21614,#17459,#17460) ;
#14494=AXIS2_PLACEMENT_3D('',#21615,#17461,#17462) ;
#16959=DIRECTION('axis',(0.,0.,1.)) ;
#16960=DIRECTION('refdir',(1.,0.,0.)) ;
#16961=DIRECTION('center_axis',(0.,0.,1.)) ;
#16962=DIRECTION('ref_axis',(1.,0.,0.)) ;
#16963=DIRECTION('center_axis',(-0.382084887170903,-0.0559079744467157,
0.922434516585792)) ;
#16964=DIRECTION('ref_axis',(0.924127230956646,-0.0231154232803137,0.381385026201834)) ;
#16965=DIRECTION('center_axis',(0.922434516585794,0.0559079744467152,-0.382084887170899)) ;
#16966=DIRECTION('ref_axis',(0.386153547971701,-0.13355165491274,0.912715395322625)) ;
#16967=DIRECTION('center_axis',(0.,0.,1.)) ;
#16968=DIRECTION('ref_axis',(1.,0.,0.)) ;
#16969=DIRECTION('center_axis',(-0.922434516585794,-0.0559079744467152,
0.382084887170899)) ;
#16970=DIRECTION('ref_axis',(0.386153547971701,-0.13355165491274,0.912715395322625)) ;
#16971=DIRECTION('center_axis',(0.922434516585793,0.0559079744467158,0.3820848871709)) ;
#16972=DIRECTION('ref_axis',(0.386153547971702,-0.13355165491274,-0.912715395322624)) ;
#16973=DIRECTION('center_axis',(0.922434516585793,0.0559079744467158,0.3820848871709)) ;
#16974=DIRECTION('ref_axis',(0.386153547971702,-0.13355165491274,-0.912715395322624)) ;
#16975=DIRECTION('center_axis',(0.,-1.,0.)) ;
#16976=DIRECTION('ref_axis',(-1.,0.,0.)) ;
#16977=DIRECTION('center_axis',(0.922434516585793,0.0559079744467158,0.3820848871709)) ;
#16978=DIRECTION('ref_axis',(0.386153547971702,-0.13355165491274,-0.912715395322624)) ;
#16979=DIRECTION('center_axis',(0.,0.,1.)) ;
#16980=DIRECTION('ref_axis',(-0.999082895817669,-0.0428178383921971,0.)) ;
#16981=DIRECTION('center_axis',(-0.922434516585793,-0.0559079744467158,
-0.3820848871709)) ;
#16982=DIRECTION('ref_axis',(0.386153547971702,-0.13355165491274,-0.912715395322624)) ;
#16983=DIRECTION('center_axis',(-0.922434516585793,-0.0559079744467158,
-0.3820848871709)) ;
#16984=DIRECTION('ref_axis',(0.386153547971702,-0.13355165491274,-0.912715395322624)) ;
#16985=DIRECTION('center_axis',(0.382084887170903,0.0559079744467153,0.922434516585792)) ;
#16986=DIRECTION('ref_axis',(0.924127230956646,-0.0231154232803136,-0.381385026201834)) ;
#16987=DIRECTION('center_axis',(0.382084887170903,0.0559079744467153,0.922434516585792)) ;
#16988=DIRECTION('ref_axis',(0.924127230956646,-0.0231154232803136,-0.381385026201834)) ;
#16989=DIRECTION('center_axis',(0.,0.,1.)) ;
#16990=DIRECTION('ref_axis',(-1.,0.,0.)) ;
#16991=DIRECTION('center_axis',(-0.382084887170903,-0.0559079744467153,
-0.922434516585792)) ;
#16992=DIRECTION('ref_axis',(0.924127230956646,-0.0231154232803136,-0.381385026201834)) ;
#16993=DIRECTION('center_axis',(-0.382084887170903,-0.0559079744467153,
-0.922434516585792)) ;
#16994=DIRECTION('ref_axis',(0.924127230956646,-0.0231154232803136,-0.381385026201834)) ;
#16995=DIRECTION('center_axis',(-0.382084887170908,0.0559079744467156,0.92243451658579)) ;
#16996=DIRECTION('ref_axis',(0.924127230956644,0.023115423280314,0.381385026201839)) ;
#16997=DIRECTION('center_axis',(-0.382084887170908,0.0559079744467156,0.92243451658579)) ;
#16998=DIRECTION('ref_axis',(0.924127230956644,0.023115423280314,0.381385026201839)) ;
#16999=DIRECTION('center_axis',(0.,0.,1.)) ;
#17000=DIRECTION('ref_axis',(-0.99908289581767,0.0428178383921882,0.)) ;
#17001=DIRECTION('center_axis',(0.382084887170908,-0.0559079744467156,-0.92243451658579)) ;
#17002=DIRECTION('ref_axis',(0.924127230956644,0.023115423280314,0.381385026201839)) ;
#17003=DIRECTION('center_axis',(0.382084887170908,-0.0559079744467156,-0.92243451658579)) ;
#17004=DIRECTION('ref_axis',(0.924127230956644,0.023115423280314,0.381385026201839)) ;
#17005=DIRECTION('center_axis',(-0.922434516585791,0.0559079744467153,0.382084887170906)) ;
#17006=DIRECTION('ref_axis',(0.386153547971708,0.133551654912737,0.912715395322622)) ;
#17007=DIRECTION('center_axis',(-0.922434516585791,0.0559079744467153,0.382084887170906)) ;
#17008=DIRECTION('ref_axis',(0.386153547971708,0.133551654912737,0.912715395322622)) ;
#17009=DIRECTION('center_axis',(0.,0.,1.)) ;
#17010=DIRECTION('ref_axis',(1.,0.,0.)) ;
#17011=DIRECTION('center_axis',(0.922434516585791,-0.0559079744467153,-0.382084887170906)) ;
#17012=DIRECTION('ref_axis',(0.386153547971708,0.133551654912737,0.912715395322622)) ;
#17013=DIRECTION('center_axis',(0.922434516585791,-0.0559079744467153,-0.382084887170906)) ;
#17014=DIRECTION('ref_axis',(0.386153547971708,0.133551654912737,0.912715395322622)) ;
#17015=DIRECTION('center_axis',(0.,-1.,0.)) ;
#17016=DIRECTION('ref_axis',(-1.,0.,0.)) ;
#17017=DIRECTION('center_axis',(0.922434516585791,-0.0559079744467153,-0.382084887170906)) ;
#17018=DIRECTION('ref_axis',(0.386153547971708,0.133551654912737,0.912715395322622)) ;
#17019=DIRECTION('center_axis',(-0.922434516585791,0.0559079744467157,-0.382084887170905)) ;
#17020=DIRECTION('ref_axis',(0.386153547971708,0.133551654912738,-0.912715395322622)) ;
#17021=DIRECTION('center_axis',(0.,0.,1.)) ;
#17022=DIRECTION('ref_axis',(1.,0.,0.)) ;
#17023=DIRECTION('center_axis',(0.922434516585791,-0.0559079744467157,0.382084887170905)) ;
#17024=DIRECTION('ref_axis',(0.386153547971708,0.133551654912738,-0.912715395322622)) ;
#17025=DIRECTION('center_axis',(-0.382084887170906,0.0559079744467161,-0.922434516585791)) ;
#17026=DIRECTION('ref_axis',(0.924127230956645,0.023115423280314,-0.381385026201837)) ;
#17027=DIRECTION('center_axis',(0.,0.,1.)) ;
#17028=DIRECTION('ref_axis',(1.,0.,0.)) ;
#17029=DIRECTION('center_axis',(0.382084887170906,-0.0559079744467161,0.922434516585791)) ;
#17030=DIRECTION('ref_axis',(0.924127230956645,0.023115423280314,-0.381385026201837)) ;
#17031=DIRECTION('center_axis',(0.382084887170903,0.0559079744467153,-0.922434516585792)) ;
#17032=DIRECTION('ref_axis',(0.924127230956646,-0.0231154232803136,0.381385026201834)) ;
#17033=DIRECTION('center_axis',(0.,0.,1.)) ;
#17034=DIRECTION('ref_axis',(1.,0.,0.)) ;
#17035=DIRECTION('center_axis',(-0.382084887170903,-0.0559079744467153,
0.922434516585792)) ;
#17036=DIRECTION('ref_axis',(0.924127230956646,-0.0231154232803136,0.381385026201834)) ;
#17037=DIRECTION('center_axis',(0.922434516585794,0.0559079744467152,-0.382084887170899)) ;
#17038=DIRECTION('ref_axis',(0.386153547971701,-0.13355165491274,0.912715395322625)) ;
#17039=DIRECTION('center_axis',(0.,0.,1.)) ;
#17040=DIRECTION('ref_axis',(1.,0.,0.)) ;
#17041=DIRECTION('center_axis',(-0.922434516585794,-0.0559079744467152,
0.382084887170899)) ;
#17042=DIRECTION('ref_axis',(0.386153547971701,-0.13355165491274,0.912715395322625)) ;
#17043=DIRECTION('center_axis',(0.922434516585793,0.0559079744467158,0.3820848871709)) ;
#17044=DIRECTION('ref_axis',(0.386153547971702,-0.13355165491274,-0.912715395322624)) ;
#17045=DIRECTION('center_axis',(0.922434516585793,0.0559079744467158,0.3820848871709)) ;
#17046=DIRECTION('ref_axis',(0.386153547971702,-0.13355165491274,-0.912715395322624)) ;
#17047=DIRECTION('center_axis',(0.,-1.,0.)) ;
#17048=DIRECTION('ref_axis',(-1.,0.,0.)) ;
#17049=DIRECTION('center_axis',(0.922434516585793,0.0559079744467158,0.3820848871709)) ;
#17050=DIRECTION('ref_axis',(0.386153547971702,-0.13355165491274,-0.912715395322624)) ;
#17051=DIRECTION('center_axis',(0.,0.,1.)) ;
#17052=DIRECTION('ref_axis',(-0.999082895817669,-0.0428178383921971,0.)) ;
#17053=DIRECTION('center_axis',(-0.922434516585793,-0.0559079744467158,
-0.3820848871709)) ;
#17054=DIRECTION('ref_axis',(0.386153547971702,-0.13355165491274,-0.912715395322624)) ;
#17055=DIRECTION('center_axis',(-0.922434516585793,-0.0559079744467158,
-0.3820848871709)) ;
#17056=DIRECTION('ref_axis',(0.386153547971702,-0.13355165491274,-0.912715395322624)) ;
#17057=DIRECTION('center_axis',(0.382084887170903,0.0559079744467153,0.922434516585792)) ;
#17058=DIRECTION('ref_axis',(0.924127230956646,-0.0231154232803136,-0.381385026201834)) ;
#17059=DIRECTION('center_axis',(0.382084887170903,0.0559079744467153,0.922434516585792)) ;
#17060=DIRECTION('ref_axis',(0.924127230956646,-0.0231154232803136,-0.381385026201834)) ;
#17061=DIRECTION('center_axis',(0.,0.,1.)) ;
#17062=DIRECTION('ref_axis',(-1.,0.,0.)) ;
#17063=DIRECTION('center_axis',(-0.382084887170903,-0.0559079744467153,
-0.922434516585792)) ;
#17064=DIRECTION('ref_axis',(0.924127230956646,-0.0231154232803136,-0.381385026201834)) ;
#17065=DIRECTION('center_axis',(-0.382084887170903,-0.0559079744467153,
-0.922434516585792)) ;
#17066=DIRECTION('ref_axis',(0.924127230956646,-0.0231154232803136,-0.381385026201834)) ;
#17067=DIRECTION('center_axis',(-0.382084887170908,0.0559079744467156,0.92243451658579)) ;
#17068=DIRECTION('ref_axis',(0.924127230956644,0.023115423280314,0.381385026201839)) ;
#17069=DIRECTION('center_axis',(-0.382084887170908,0.0559079744467156,0.92243451658579)) ;
#17070=DIRECTION('ref_axis',(0.924127230956644,0.023115423280314,0.381385026201839)) ;
#17071=DIRECTION('center_axis',(0.,0.,1.)) ;
#17072=DIRECTION('ref_axis',(-0.99908289581767,0.0428178383921882,0.)) ;
#17073=DIRECTION('center_axis',(0.382084887170908,-0.0559079744467156,-0.92243451658579)) ;
#17074=DIRECTION('ref_axis',(0.924127230956644,0.023115423280314,0.381385026201839)) ;
#17075=DIRECTION('center_axis',(0.382084887170908,-0.0559079744467156,-0.92243451658579)) ;
#17076=DIRECTION('ref_axis',(0.924127230956644,0.023115423280314,0.381385026201839)) ;
#17077=DIRECTION('center_axis',(-0.922434516585791,0.0559079744467157,0.382084887170905)) ;
#17078=DIRECTION('ref_axis',(0.386153547971708,0.133551654912738,0.912715395322622)) ;
#17079=DIRECTION('center_axis',(-0.922434516585791,0.0559079744467157,0.382084887170905)) ;
#17080=DIRECTION('ref_axis',(0.386153547971708,0.133551654912738,0.912715395322622)) ;
#17081=DIRECTION('center_axis',(0.,0.,1.)) ;
#17082=DIRECTION('ref_axis',(1.,0.,0.)) ;
#17083=DIRECTION('center_axis',(0.922434516585791,-0.0559079744467157,-0.382084887170905)) ;
#17084=DIRECTION('ref_axis',(0.386153547971708,0.133551654912738,0.912715395322622)) ;
#17085=DIRECTION('center_axis',(0.922434516585791,-0.0559079744467157,-0.382084887170905)) ;
#17086=DIRECTION('ref_axis',(0.386153547971708,0.133551654912738,0.912715395322622)) ;
#17087=DIRECTION('center_axis',(0.,-1.,0.)) ;
#17088=DIRECTION('ref_axis',(-1.,0.,0.)) ;
#17089=DIRECTION('center_axis',(0.922434516585791,-0.0559079744467157,-0.382084887170905)) ;
#17090=DIRECTION('ref_axis',(0.386153547971708,0.133551654912738,0.912715395322622)) ;
#17091=DIRECTION('center_axis',(-0.922434516585791,0.0559079744467157,-0.382084887170905)) ;
#17092=DIRECTION('ref_axis',(0.386153547971708,0.133551654912738,-0.912715395322622)) ;
#17093=DIRECTION('center_axis',(0.,0.,1.)) ;
#17094=DIRECTION('ref_axis',(1.,0.,0.)) ;
#17095=DIRECTION('center_axis',(0.922434516585791,-0.0559079744467157,0.382084887170905)) ;
#17096=DIRECTION('ref_axis',(0.386153547971708,0.133551654912738,-0.912715395322622)) ;
#17097=DIRECTION('center_axis',(-0.382084887170905,0.0559079744467153,-0.922434516585791)) ;
#17098=DIRECTION('ref_axis',(0.924127230956645,0.0231154232803137,-0.381385026201837)) ;
#17099=DIRECTION('center_axis',(0.,0.,1.)) ;
#17100=DIRECTION('ref_axis',(1.,0.,0.)) ;
#17101=DIRECTION('center_axis',(0.382084887170905,-0.0559079744467153,0.922434516585791)) ;
#17102=DIRECTION('ref_axis',(0.924127230956645,0.0231154232803137,-0.381385026201837)) ;
#17103=DIRECTION('center_axis',(0.382084887170903,0.0559079744467153,-0.922434516585792)) ;
#17104=DIRECTION('ref_axis',(0.924127230956646,-0.0231154232803136,0.381385026201834)) ;
#17105=DIRECTION('center_axis',(0.,0.,1.)) ;
#17106=DIRECTION('ref_axis',(1.,0.,0.)) ;
#17107=DIRECTION('center_axis',(-0.382084887170903,-0.0559079744467153,
0.922434516585792)) ;
#17108=DIRECTION('ref_axis',(0.924127230956646,-0.0231154232803136,0.381385026201834)) ;
#17109=DIRECTION('center_axis',(0.922434516585793,0.0559079744467162,-0.3820848871709)) ;
#17110=DIRECTION('ref_axis',(0.386153547971703,-0.133551654912741,0.912715395322624)) ;
#17111=DIRECTION('center_axis',(0.,0.,1.)) ;
#17112=DIRECTION('ref_axis',(1.,0.,0.)) ;
#17113=DIRECTION('center_axis',(-0.922434516585793,-0.0559079744467162,
0.3820848871709)) ;
#17114=DIRECTION('ref_axis',(0.386153547971703,-0.133551654912741,0.912715395322624)) ;
#17115=DIRECTION('center_axis',(0.922434516585794,0.0559079744467152,0.382084887170899)) ;
#17116=DIRECTION('ref_axis',(0.386153547971701,-0.13355165491274,-0.912715395322625)) ;
#17117=DIRECTION('center_axis',(0.922434516585794,0.0559079744467152,0.382084887170899)) ;
#17118=DIRECTION('ref_axis',(0.386153547971701,-0.13355165491274,-0.912715395322625)) ;
#17119=DIRECTION('center_axis',(0.,-1.,0.)) ;
#17120=DIRECTION('ref_axis',(-1.,0.,0.)) ;
#17121=DIRECTION('center_axis',(0.922434516585794,0.0559079744467152,0.382084887170899)) ;
#17122=DIRECTION('ref_axis',(0.386153547971701,-0.13355165491274,-0.912715395322625)) ;
#17123=DIRECTION('center_axis',(0.,0.,1.)) ;
#17124=DIRECTION('ref_axis',(-0.99908289581767,-0.0428178383921882,0.)) ;
#17125=DIRECTION('center_axis',(-0.922434516585794,-0.0559079744467152,
-0.382084887170899)) ;
#17126=DIRECTION('ref_axis',(0.386153547971701,-0.13355165491274,-0.912715395322625)) ;
#17127=DIRECTION('center_axis',(-0.922434516585794,-0.0559079744467152,
-0.382084887170899)) ;
#17128=DIRECTION('ref_axis',(0.386153547971701,-0.13355165491274,-0.912715395322625)) ;
#17129=DIRECTION('center_axis',(0.382084887170903,0.0559079744467153,0.922434516585792)) ;
#17130=DIRECTION('ref_axis',(0.924127230956646,-0.0231154232803136,-0.381385026201834)) ;
#17131=DIRECTION('center_axis',(0.382084887170903,0.0559079744467153,0.922434516585792)) ;
#17132=DIRECTION('ref_axis',(0.924127230956646,-0.0231154232803136,-0.381385026201834)) ;
#17133=DIRECTION('center_axis',(0.,0.,1.)) ;
#17134=DIRECTION('ref_axis',(-1.,0.,0.)) ;
#17135=DIRECTION('center_axis',(-0.382084887170903,-0.0559079744467153,
-0.922434516585792)) ;
#17136=DIRECTION('ref_axis',(0.924127230956646,-0.0231154232803136,-0.381385026201834)) ;
#17137=DIRECTION('center_axis',(-0.382084887170903,-0.0559079744467153,
-0.922434516585792)) ;
#17138=DIRECTION('ref_axis',(0.924127230956646,-0.0231154232803136,-0.381385026201834)) ;
#17139=DIRECTION('center_axis',(-0.382084887170908,0.0559079744467156,0.92243451658579)) ;
#17140=DIRECTION('ref_axis',(0.924127230956644,0.023115423280314,0.381385026201839)) ;
#17141=DIRECTION('center_axis',(-0.382084887170908,0.0559079744467156,0.92243451658579)) ;
#17142=DIRECTION('ref_axis',(0.924127230956644,0.023115423280314,0.381385026201839)) ;
#17143=DIRECTION('center_axis',(0.,0.,1.)) ;
#17144=DIRECTION('ref_axis',(-0.99908289581767,0.0428178383921882,0.)) ;
#17145=DIRECTION('center_axis',(0.382084887170908,-0.0559079744467156,-0.92243451658579)) ;
#17146=DIRECTION('ref_axis',(0.924127230956644,0.023115423280314,0.381385026201839)) ;
#17147=DIRECTION('center_axis',(0.382084887170908,-0.0559079744467156,-0.92243451658579)) ;
#17148=DIRECTION('ref_axis',(0.924127230956644,0.023115423280314,0.381385026201839)) ;
#17149=DIRECTION('center_axis',(-0.922434516585791,0.0559079744467157,0.382084887170905)) ;
#17150=DIRECTION('ref_axis',(0.386153547971708,0.133551654912738,0.912715395322622)) ;
#17151=DIRECTION('center_axis',(-0.922434516585791,0.0559079744467157,0.382084887170905)) ;
#17152=DIRECTION('ref_axis',(0.386153547971708,0.133551654912738,0.912715395322622)) ;
#17153=DIRECTION('center_axis',(0.,0.,1.)) ;
#17154=DIRECTION('ref_axis',(1.,0.,0.)) ;
#17155=DIRECTION('center_axis',(0.922434516585791,-0.0559079744467157,-0.382084887170905)) ;
#17156=DIRECTION('ref_axis',(0.386153547971708,0.133551654912738,0.912715395322622)) ;
#17157=DIRECTION('center_axis',(0.922434516585791,-0.0559079744467157,-0.382084887170905)) ;
#17158=DIRECTION('ref_axis',(0.386153547971708,0.133551654912738,0.912715395322622)) ;
#17159=DIRECTION('center_axis',(0.,-1.,0.)) ;
#17160=DIRECTION('ref_axis',(-1.,0.,0.)) ;
#17161=DIRECTION('center_axis',(0.922434516585791,-0.0559079744467157,-0.382084887170905)) ;
#17162=DIRECTION('ref_axis',(0.386153547971708,0.133551654912738,0.912715395322622)) ;
#17163=DIRECTION('center_axis',(-0.922434516585791,0.0559079744467157,-0.382084887170905)) ;
#17164=DIRECTION('ref_axis',(0.386153547971708,0.133551654912738,-0.912715395322622)) ;
#17165=DIRECTION('center_axis',(0.,0.,1.)) ;
#17166=DIRECTION('ref_axis',(1.,0.,0.)) ;
#17167=DIRECTION('center_axis',(0.922434516585791,-0.0559079744467157,0.382084887170905)) ;
#17168=DIRECTION('ref_axis',(0.386153547971708,0.133551654912738,-0.912715395322622)) ;
#17169=DIRECTION('center_axis',(-0.382084887170906,0.0559079744467155,-0.922434516585791)) ;
#17170=DIRECTION('ref_axis',(0.924127230956645,0.0231154232803138,-0.381385026201837)) ;
#17171=DIRECTION('center_axis',(0.,0.,1.)) ;
#17172=DIRECTION('ref_axis',(1.,0.,0.)) ;
#17173=DIRECTION('center_axis',(0.382084887170906,-0.0559079744467155,0.922434516585791)) ;
#17174=DIRECTION('ref_axis',(0.924127230956645,0.0231154232803138,-0.381385026201837)) ;
#17175=DIRECTION('center_axis',(0.382084887170903,0.0559079744467153,-0.922434516585792)) ;
#17176=DIRECTION('ref_axis',(0.924127230956646,-0.0231154232803136,0.381385026201834)) ;
#17177=DIRECTION('center_axis',(0.,0.,1.)) ;
#17178=DIRECTION('ref_axis',(1.,0.,0.)) ;
#17179=DIRECTION('center_axis',(-0.382084887170903,-0.0559079744467153,
0.922434516585792)) ;
#17180=DIRECTION('ref_axis',(0.924127230956646,-0.0231154232803136,0.381385026201834)) ;
#17181=DIRECTION('center_axis',(0.922434516585793,0.0559079744467156,-0.3820848871709)) ;
#17182=DIRECTION('ref_axis',(0.386153547971702,-0.13355165491274,0.912715395322624)) ;
#17183=DIRECTION('center_axis',(0.,0.,1.)) ;
#17184=DIRECTION('ref_axis',(1.,0.,0.)) ;
#17185=DIRECTION('center_axis',(-0.922434516585793,-0.0559079744467156,
0.3820848871709)) ;
#17186=DIRECTION('ref_axis',(0.386153547971702,-0.13355165491274,0.912715395322624)) ;
#17187=DIRECTION('center_axis',(0.922434516585794,0.0559079744467156,0.382084887170899)) ;
#17188=DIRECTION('ref_axis',(0.386153547971701,-0.133551654912741,-0.912715395322625)) ;
#17189=DIRECTION('center_axis',(0.922434516585794,0.0559079744467156,0.382084887170899)) ;
#17190=DIRECTION('ref_axis',(0.386153547971701,-0.133551654912741,-0.912715395322625)) ;
#17191=DIRECTION('center_axis',(0.,-1.,0.)) ;
#17192=DIRECTION('ref_axis',(-1.,0.,0.)) ;
#17193=DIRECTION('center_axis',(0.922434516585794,0.0559079744467156,0.382084887170899)) ;
#17194=DIRECTION('ref_axis',(0.386153547971701,-0.133551654912741,-0.912715395322625)) ;
#17195=DIRECTION('center_axis',(0.,0.,1.)) ;
#17196=DIRECTION('ref_axis',(-0.99908289581767,-0.0428178383921882,0.)) ;
#17197=DIRECTION('center_axis',(-0.922434516585794,-0.0559079744467156,
-0.382084887170899)) ;
#17198=DIRECTION('ref_axis',(0.386153547971701,-0.133551654912741,-0.912715395322625)) ;
#17199=DIRECTION('center_axis',(-0.922434516585794,-0.0559079744467156,
-0.382084887170899)) ;
#17200=DIRECTION('ref_axis',(0.386153547971701,-0.133551654912741,-0.912715395322625)) ;
#17201=DIRECTION('center_axis',(0.382084887170903,0.0559079744467155,0.922434516585792)) ;
#17202=DIRECTION('ref_axis',(0.924127230956646,-0.0231154232803136,-0.381385026201834)) ;
#17203=DIRECTION('center_axis',(0.382084887170903,0.0559079744467155,0.922434516585792)) ;
#17204=DIRECTION('ref_axis',(0.924127230956646,-0.0231154232803136,-0.381385026201834)) ;
#17205=DIRECTION('center_axis',(0.,0.,1.)) ;
#17206=DIRECTION('ref_axis',(-1.,8.88178419700128E-15,0.)) ;
#17207=DIRECTION('center_axis',(-0.382084887170903,-0.0559079744467155,
-0.922434516585792)) ;
#17208=DIRECTION('ref_axis',(0.924127230956646,-0.0231154232803136,-0.381385026201834)) ;
#17209=DIRECTION('center_axis',(-0.382084887170903,-0.0559079744467155,
-0.922434516585792)) ;
#17210=DIRECTION('ref_axis',(0.924127230956646,-0.0231154232803136,-0.381385026201834)) ;
#17211=DIRECTION('center_axis',(-0.382084887170906,0.0559079744467155,0.922434516585791)) ;
#17212=DIRECTION('ref_axis',(0.924127230956645,0.0231154232803138,0.381385026201837)) ;
#17213=DIRECTION('center_axis',(-0.382084887170906,0.0559079744467155,0.922434516585791)) ;
#17214=DIRECTION('ref_axis',(0.924127230956645,0.0231154232803138,0.381385026201837)) ;
#17215=DIRECTION('center_axis',(0.,0.,1.)) ;
#17216=DIRECTION('ref_axis',(-0.99908289581767,0.0428178383921793,0.)) ;
#17217=DIRECTION('center_axis',(0.382084887170906,-0.0559079744467155,-0.922434516585791)) ;
#17218=DIRECTION('ref_axis',(0.924127230956645,0.0231154232803138,0.381385026201837)) ;
#17219=DIRECTION('center_axis',(0.382084887170906,-0.0559079744467155,-0.922434516585791)) ;
#17220=DIRECTION('ref_axis',(0.924127230956645,0.0231154232803138,0.381385026201837)) ;
#17221=DIRECTION('center_axis',(-0.922434516585792,0.0559079744467155,0.382084887170904)) ;
#17222=DIRECTION('ref_axis',(0.386153547971707,0.133551654912738,0.912715395322623)) ;
#17223=DIRECTION('center_axis',(-0.922434516585792,0.0559079744467155,0.382084887170904)) ;
#17224=DIRECTION('ref_axis',(0.386153547971707,0.133551654912738,0.912715395322623)) ;
#17225=DIRECTION('center_axis',(0.,0.,1.)) ;
#17226=DIRECTION('ref_axis',(1.,0.,0.)) ;
#17227=DIRECTION('center_axis',(0.922434516585792,-0.0559079744467155,-0.382084887170904)) ;
#17228=DIRECTION('ref_axis',(0.386153547971707,0.133551654912738,0.912715395322623)) ;
#17229=DIRECTION('center_axis',(0.922434516585792,-0.0559079744467155,-0.382084887170904)) ;
#17230=DIRECTION('ref_axis',(0.386153547971707,0.133551654912738,0.912715395322623)) ;
#17231=DIRECTION('center_axis',(0.,-1.,0.)) ;
#17232=DIRECTION('ref_axis',(-1.,0.,0.)) ;
#17233=DIRECTION('center_axis',(0.922434516585792,-0.0559079744467155,-0.382084887170904)) ;
#17234=DIRECTION('ref_axis',(0.386153547971707,0.133551654912738,0.912715395322623)) ;
#17235=DIRECTION('center_axis',(-0.922434516585791,0.0559079744467157,-0.382084887170905)) ;
#17236=DIRECTION('ref_axis',(0.386153547971708,0.133551654912738,-0.912715395322622)) ;
#17237=DIRECTION('center_axis',(0.,0.,1.)) ;
#17238=DIRECTION('ref_axis',(1.,0.,0.)) ;
#17239=DIRECTION('center_axis',(0.922434516585791,-0.0559079744467157,0.382084887170905)) ;
#17240=DIRECTION('ref_axis',(0.386153547971708,0.133551654912738,-0.912715395322622)) ;
#17241=DIRECTION('center_axis',(-0.382084887170906,0.0559079744467155,-0.922434516585791)) ;
#17242=DIRECTION('ref_axis',(0.924127230956645,0.0231154232803138,-0.381385026201837)) ;
#17243=DIRECTION('center_axis',(0.382084887170903,0.0559079744467157,-0.922434516585792)) ;
#17244=DIRECTION('ref_axis',(0.924127230956646,-0.0231154232803137,0.381385026201834)) ;
#17245=DIRECTION('center_axis',(0.382084887170903,0.0559079744467157,-0.922434516585792)) ;
#17246=DIRECTION('ref_axis',(0.924127230956646,-0.0231154232803137,0.381385026201834)) ;
#17247=DIRECTION('',(-0.382084887170903,-0.0559079744467157,0.922434516585792)) ;
#17248=DIRECTION('center_axis',(-0.705811580947695,-0.0604981355097965,
0.705811580947745)) ;
#17249=DIRECTION('ref_axis',(0.707106781186573,-1.76822503816994E-14,0.707106781186522)) ;
#17250=DIRECTION('center_axis',(-0.705811580947695,-0.0604981355097965,
0.705811580947745)) ;
#17251=DIRECTION('ref_axis',(0.707106781186573,-1.76822503816994E-14,0.707106781186522)) ;
#17252=DIRECTION('center_axis',(-0.705811580947695,-0.0604981355097965,
0.705811580947745)) ;
#17253=DIRECTION('ref_axis',(0.707106781186573,-1.76822503816994E-14,0.707106781186522)) ;
#17254=DIRECTION('center_axis',(0.382084887170903,0.0559079744467157,-0.922434516585792)) ;
#17255=DIRECTION('ref_axis',(0.924127230956646,-0.0231154232803137,0.381385026201834)) ;
#17256=DIRECTION('center_axis',(0.922434516585794,0.0559079744467152,-0.382084887170899)) ;
#17257=DIRECTION('ref_axis',(0.386153547971701,-0.13355165491274,0.912715395322625)) ;
#17258=DIRECTION('',(-0.922434516585794,-0.0559079744467152,0.382084887170899)) ;
#17259=DIRECTION('center_axis',(-0.99816831025626,-0.0604981355098033,-1.24140640981796E-16)) ;
#17260=DIRECTION('ref_axis',(-3.40659855495112E-17,-1.13820469365426E-15,
1.)) ;
#17261=DIRECTION('center_axis',(-0.99816831025626,-0.0604981355098033,-1.24140640981796E-16)) ;
#17262=DIRECTION('ref_axis',(-3.40659855495112E-17,-1.13820469365426E-15,
1.)) ;
#17263=DIRECTION('center_axis',(0.922434516585793,0.0559079744467158,0.3820848871709)) ;
#17264=DIRECTION('ref_axis',(0.386153547971702,-0.13355165491274,-0.912715395322624)) ;
#17265=DIRECTION('',(-0.922434516585793,-0.0559079744467158,-0.3820848871709)) ;
#17266=DIRECTION('center_axis',(-0.705811580947751,-0.0604981355097965,
-0.705811580947687)) ;
#17267=DIRECTION('ref_axis',(0.707106781186515,1.77143124857461E-14,-0.70710678118658)) ;
#17268=DIRECTION('center_axis',(0.382084887170903,0.0559079744467153,0.922434516585792)) ;
#17269=DIRECTION('ref_axis',(0.924127230956646,-0.0231154232803136,-0.381385026201834)) ;
#17270=DIRECTION('',(-0.382084887170903,-0.0559079744467153,-0.922434516585792)) ;
#17271=DIRECTION('center_axis',(3.28955978897023E-14,-0.0604981355098033,
-0.99816831025626)) ;
#17272=DIRECTION('ref_axis',(1.,1.99586597690074E-15,3.28957187518098E-14)) ;
#17273=DIRECTION('center_axis',(-0.382084887170908,0.0559079744467156,0.92243451658579)) ;
#17274=DIRECTION('ref_axis',(0.924127230956644,0.023115423280314,0.381385026201839)) ;
#17275=DIRECTION('',(0.382084887170908,-0.0559079744467156,-0.92243451658579)) ;
#17276=DIRECTION('center_axis',(0.705811580947711,-0.0604981355097965,-0.705811580947728)) ;
#17277=DIRECTION('ref_axis',(0.707106781186557,1.85078495608992E-14,0.707106781186538)) ;
#17278=DIRECTION('center_axis',(-0.922434516585791,0.0559079744467153,0.382084887170906)) ;
#17279=DIRECTION('ref_axis',(0.386153547971708,0.133551654912737,0.912715395322622)) ;
#17280=DIRECTION('',(0.922434516585791,-0.0559079744467153,-0.382084887170905)) ;
#17281=DIRECTION('center_axis',(0.99816831025626,-0.0604981355098033,-3.28955978897028E-14)) ;
#17282=DIRECTION('ref_axis',(3.29408060856262E-14,2.08403676302894E-16,
1.)) ;
#17283=DIRECTION('center_axis',(0.99816831025626,-0.0604981355098033,-3.28955978897028E-14)) ;
#17284=DIRECTION('ref_axis',(3.29408060856262E-14,2.08403676302894E-16,
1.)) ;
#17285=DIRECTION('center_axis',(-0.922434516585791,0.0559079744467157,-0.382084887170905)) ;
#17286=DIRECTION('ref_axis',(0.386153547971708,0.133551654912738,-0.912715395322622)) ;
#17287=DIRECTION('',(0.922434516585791,-0.0559079744467157,0.382084887170906)) ;
#17288=DIRECTION('center_axis',(0.705811580947752,-0.0604981355097965,0.705811580947687)) ;
#17289=DIRECTION('ref_axis',(0.707106781186515,-1.71051325088607E-14,-0.70710678118658)) ;
#17290=DIRECTION('center_axis',(0.705811580947752,-0.0604981355097965,0.705811580947687)) ;
#17291=DIRECTION('ref_axis',(0.707106781186515,-1.71051325088607E-14,-0.70710678118658)) ;
#17292=DIRECTION('center_axis',(0.705811580947752,-0.0604981355097965,0.705811580947687)) ;
#17293=DIRECTION('ref_axis',(0.707106781186515,-1.71051325088607E-14,-0.70710678118658)) ;
#17294=DIRECTION('center_axis',(-0.382084887170906,0.0559079744467161,-0.922434516585791)) ;
#17295=DIRECTION('ref_axis',(0.924127230956645,0.023115423280314,-0.381385026201837)) ;
#17296=DIRECTION('',(0.382084887170905,-0.0559079744467161,0.922434516585791)) ;
#17297=DIRECTION('center_axis',(0.,-0.0604981355098033,0.99816831025626)) ;
#17298=DIRECTION('ref_axis',(1.,0.,0.)) ;
#17299=DIRECTION('center_axis',(0.,-0.0604981355098033,0.99816831025626)) ;
#17300=DIRECTION('ref_axis',(1.,0.,0.)) ;
#17301=DIRECTION('center_axis',(0.382084887170903,0.0559079744467153,-0.922434516585792)) ;
#17302=DIRECTION('ref_axis',(0.924127230956646,-0.0231154232803136,0.381385026201834)) ;
#17303=DIRECTION('',(-0.382084887170903,-0.0559079744467153,0.922434516585792)) ;
#17304=DIRECTION('center_axis',(-0.705811580947711,-0.0604981355097965,
0.705811580947728)) ;
#17305=DIRECTION('ref_axis',(0.707106781186557,-1.80750111562701E-14,0.707106781186538)) ;
#17306=DIRECTION('center_axis',(-0.705811580947711,-0.0604981355097965,
0.705811580947728)) ;
#17307=DIRECTION('ref_axis',(0.707106781186557,-1.80750111562701E-14,0.707106781186538)) ;
#17308=DIRECTION('center_axis',(-0.705811580947711,-0.0604981355097965,
0.705811580947728)) ;
#17309=DIRECTION('ref_axis',(0.707106781186557,-1.80750111562701E-14,0.707106781186538)) ;
#17310=DIRECTION('center_axis',(0.922434516585794,0.0559079744467152,-0.382084887170899)) ;
#17311=DIRECTION('ref_axis',(0.386153547971701,-0.13355165491274,0.912715395322625)) ;
#17312=DIRECTION('',(-0.922434516585794,-0.0559079744467152,0.382084887170899)) ;
#17313=DIRECTION('center_axis',(-0.99816831025626,-0.0604981355098033,-1.24140640981796E-16)) ;
#17314=DIRECTION('ref_axis',(-3.40659855495112E-17,-1.13820469365426E-15,
1.)) ;
#17315=DIRECTION('center_axis',(-0.99816831025626,-0.0604981355098033,-1.24140640981796E-16)) ;
#17316=DIRECTION('ref_axis',(-3.40659855495112E-17,-1.13820469365426E-15,
1.)) ;
#17317=DIRECTION('center_axis',(0.922434516585793,0.0559079744467158,0.3820848871709)) ;
#17318=DIRECTION('ref_axis',(0.386153547971702,-0.13355165491274,-0.912715395322624)) ;
#17319=DIRECTION('',(-0.922434516585793,-0.0559079744467158,-0.3820848871709)) ;
#17320=DIRECTION('center_axis',(-0.705811580947751,-0.0604981355097965,
-0.705811580947687)) ;
#17321=DIRECTION('ref_axis',(0.707106781186515,1.77143124857461E-14,-0.70710678118658)) ;
#17322=DIRECTION('center_axis',(0.382084887170903,0.0559079744467153,0.922434516585792)) ;
#17323=DIRECTION('ref_axis',(0.924127230956646,-0.0231154232803136,-0.381385026201834)) ;
#17324=DIRECTION('',(-0.382084887170903,-0.0559079744467153,-0.922434516585792)) ;
#17325=DIRECTION('center_axis',(3.28955978897023E-14,-0.0604981355098033,
-0.99816831025626)) ;
#17326=DIRECTION('ref_axis',(1.,1.99586597690074E-15,3.28957187518098E-14)) ;
#17327=DIRECTION('center_axis',(-0.382084887170908,0.0559079744467156,0.92243451658579)) ;
#17328=DIRECTION('ref_axis',(0.924127230956644,0.023115423280314,0.381385026201839)) ;
#17329=DIRECTION('',(0.382084887170908,-0.0559079744467156,-0.92243451658579)) ;
#17330=DIRECTION('center_axis',(0.705811580947711,-0.0604981355097965,-0.705811580947728)) ;
#17331=DIRECTION('ref_axis',(0.707106781186557,1.85078495608992E-14,0.707106781186538)) ;
#17332=DIRECTION('center_axis',(-0.922434516585791,0.0559079744467157,0.382084887170905)) ;
#17333=DIRECTION('ref_axis',(0.386153547971708,0.133551654912738,0.912715395322622)) ;
#17334=DIRECTION('',(0.922434516585791,-0.0559079744467157,-0.382084887170906)) ;
#17335=DIRECTION('center_axis',(0.99816831025626,-0.0604981355098033,-3.28955978897028E-14)) ;
#17336=DIRECTION('ref_axis',(3.30470118052806E-14,9.13769965328074E-16,
1.)) ;
#17337=DIRECTION('center_axis',(0.99816831025626,-0.0604981355098033,-3.28955978897028E-14)) ;
#17338=DIRECTION('ref_axis',(3.30470118052806E-14,9.13769965328074E-16,
1.)) ;
#17339=DIRECTION('center_axis',(-0.922434516585791,0.0559079744467157,-0.382084887170905)) ;
#17340=DIRECTION('ref_axis',(0.386153547971708,0.133551654912738,-0.912715395322622)) ;
#17341=DIRECTION('',(0.922434516585791,-0.0559079744467157,0.382084887170906)) ;
#17342=DIRECTION('center_axis',(0.705811580947752,-0.0604981355097965,0.705811580947687)) ;
#17343=DIRECTION('ref_axis',(0.707106781186515,-1.71532256649306E-14,-0.70710678118658)) ;
#17344=DIRECTION('center_axis',(0.705811580947752,-0.0604981355097965,0.705811580947687)) ;
#17345=DIRECTION('ref_axis',(0.707106781186515,-1.71532256649306E-14,-0.70710678118658)) ;
#17346=DIRECTION('center_axis',(0.705811580947752,-0.0604981355097965,0.705811580947687)) ;
#17347=DIRECTION('ref_axis',(0.707106781186515,-1.71532256649306E-14,-0.70710678118658)) ;
#17348=DIRECTION('center_axis',(-0.382084887170905,0.0559079744467153,-0.922434516585791)) ;
#17349=DIRECTION('ref_axis',(0.924127230956645,0.0231154232803137,-0.381385026201837)) ;
#17350=DIRECTION('',(0.382084887170906,-0.0559079744467153,0.922434516585791)) ;
#17351=DIRECTION('center_axis',(0.,-0.0604981355098033,0.99816831025626)) ;
#17352=DIRECTION('ref_axis',(1.,-4.00776300582483E-18,6.41242080931973E-17)) ;
#17353=DIRECTION('center_axis',(0.,-0.0604981355098033,0.99816831025626)) ;
#17354=DIRECTION('ref_axis',(1.,-4.00776300582483E-18,6.41242080931973E-17)) ;
#17355=DIRECTION('center_axis',(0.382084887170903,0.0559079744467153,-0.922434516585792)) ;
#17356=DIRECTION('ref_axis',(0.924127230956646,-0.0231154232803136,0.381385026201834)) ;
#17357=DIRECTION('',(-0.382084887170903,-0.0559079744467153,0.922434516585792)) ;
#17358=DIRECTION('center_axis',(-0.705811580947719,-0.0604981355097965,
0.70581158094772)) ;
#17359=DIRECTION('ref_axis',(0.707106781186549,-1.87883929713068E-14,0.707106781186546)) ;
#17360=DIRECTION('center_axis',(-0.705811580947719,-0.0604981355097965,
0.70581158094772)) ;
#17361=DIRECTION('ref_axis',(0.707106781186549,-1.87883929713068E-14,0.707106781186546)) ;
#17362=DIRECTION('center_axis',(-0.705811580947719,-0.0604981355097965,
0.70581158094772)) ;
#17363=DIRECTION('ref_axis',(0.707106781186549,-1.87883929713068E-14,0.707106781186546)) ;
#17364=DIRECTION('center_axis',(0.922434516585793,0.0559079744467162,-0.3820848871709)) ;
#17365=DIRECTION('ref_axis',(0.386153547971703,-0.133551654912741,0.912715395322624)) ;
#17366=DIRECTION('',(-0.922434516585793,-0.0559079744467162,0.3820848871709)) ;
#17367=DIRECTION('center_axis',(-0.99816831025626,-0.0604981355098033,-2.48281281963583E-16)) ;
#17368=DIRECTION('ref_axis',(-3.10601632951425E-17,-4.45663246247722E-15,
1.)) ;
#17369=DIRECTION('center_axis',(-0.99816831025626,-0.0604981355098033,-2.48281281963583E-16)) ;
#17370=DIRECTION('ref_axis',(-3.10601632951425E-17,-4.45663246247722E-15,
1.)) ;
#17371=DIRECTION('center_axis',(0.922434516585794,0.0559079744467152,0.382084887170899)) ;
#17372=DIRECTION('ref_axis',(0.386153547971701,-0.13355165491274,-0.912715395322625)) ;
#17373=DIRECTION('',(-0.922434516585794,-0.0559079744467152,-0.382084887170899)) ;
#17374=DIRECTION('center_axis',(-0.70581158094776,-0.0604981355097965,-0.705811580947679)) ;
#17375=DIRECTION('ref_axis',(0.707106781186506,1.55982136186706E-14,-0.707106781186589)) ;
#17376=DIRECTION('center_axis',(0.382084887170903,0.0559079744467153,0.922434516585792)) ;
#17377=DIRECTION('ref_axis',(0.924127230956646,-0.0231154232803136,-0.381385026201834)) ;
#17378=DIRECTION('',(-0.382084887170903,-0.0559079744467153,-0.922434516585792)) ;
#17379=DIRECTION('center_axis',(3.28955978897023E-14,-0.0604981355098033,
-0.99816831025626)) ;
#17380=DIRECTION('ref_axis',(1.,1.99586597690074E-15,3.28957187518098E-14)) ;
#17381=DIRECTION('center_axis',(-0.382084887170908,0.0559079744467156,0.92243451658579)) ;
#17382=DIRECTION('ref_axis',(0.924127230956644,0.023115423280314,0.381385026201839)) ;
#17383=DIRECTION('',(0.382084887170908,-0.0559079744467156,-0.92243451658579)) ;
#17384=DIRECTION('center_axis',(0.705811580947711,-0.0604981355097965,-0.705811580947728)) ;
#17385=DIRECTION('ref_axis',(0.707106781186557,1.85078495608992E-14,0.707106781186538)) ;
#17386=DIRECTION('center_axis',(-0.922434516585791,0.0559079744467157,0.382084887170905)) ;
#17387=DIRECTION('ref_axis',(0.386153547971708,0.133551654912738,0.912715395322622)) ;
#17388=DIRECTION('',(0.922434516585791,-0.0559079744467157,-0.382084887170906)) ;
#17389=DIRECTION('center_axis',(0.99816831025626,-0.0604981355098033,-3.28955978897028E-14)) ;
#17390=DIRECTION('ref_axis',(3.30650467388068E-14,1.04201838151447E-15,
1.)) ;
#17391=DIRECTION('center_axis',(0.99816831025626,-0.0604981355098033,-3.28955978897028E-14)) ;
#17392=DIRECTION('ref_axis',(3.30650467388068E-14,1.04201838151447E-15,
1.)) ;
#17393=DIRECTION('center_axis',(-0.922434516585791,0.0559079744467157,-0.382084887170905)) ;
#17394=DIRECTION('ref_axis',(0.386153547971708,0.133551654912738,-0.912715395322622)) ;
#17395=DIRECTION('',(0.922434516585791,-0.0559079744467157,0.382084887170906)) ;
#17396=DIRECTION('center_axis',(0.70581158094776,-0.0604981355097964,0.705811580947679)) ;
#17397=DIRECTION('ref_axis',(0.707106781186506,-1.66081698961385E-14,-0.707106781186589)) ;
#17398=DIRECTION('center_axis',(0.70581158094776,-0.0604981355097964,0.705811580947679)) ;
#17399=DIRECTION('ref_axis',(0.707106781186506,-1.66081698961385E-14,-0.707106781186589)) ;
#17400=DIRECTION('center_axis',(0.70581158094776,-0.0604981355097964,0.705811580947679)) ;
#17401=DIRECTION('ref_axis',(0.707106781186506,-1.66081698961385E-14,-0.707106781186589)) ;
#17402=DIRECTION('center_axis',(-0.382084887170906,0.0559079744467155,-0.922434516585791)) ;
#17403=DIRECTION('ref_axis',(0.924127230956645,0.0231154232803138,-0.381385026201837)) ;
#17404=DIRECTION('',(0.382084887170905,-0.0559079744467155,0.922434516585791)) ;
#17405=DIRECTION('center_axis',(-1.24140640981796E-16,-0.0604981355098033,
0.99816831025626)) ;
#17406=DIRECTION('ref_axis',(1.,-1.20232890174745E-17,1.92372624279592E-16)) ;
#17407=DIRECTION('center_axis',(-1.24140640981796E-16,-0.0604981355098033,
0.99816831025626)) ;
#17408=DIRECTION('ref_axis',(1.,-1.20232890174745E-17,1.92372624279592E-16)) ;
#17409=DIRECTION('center_axis',(0.382084887170903,0.0559079744467153,-0.922434516585792)) ;
#17410=DIRECTION('ref_axis',(0.924127230956646,-0.0231154232803136,0.381385026201834)) ;
#17411=DIRECTION('',(-0.382084887170903,-0.0559079744467153,0.922434516585792)) ;
#17412=DIRECTION('center_axis',(-0.705811580947719,-0.0604981355097965,
0.70581158094772)) ;
#17413=DIRECTION('ref_axis',(0.707106781186549,-1.88044240233301E-14,0.707106781186546)) ;
#17414=DIRECTION('center_axis',(-0.705811580947719,-0.0604981355097965,
0.70581158094772)) ;
#17415=DIRECTION('ref_axis',(0.707106781186549,-1.88044240233301E-14,0.707106781186546)) ;
#17416=DIRECTION('center_axis',(-0.705811580947719,-0.0604981355097965,
0.70581158094772)) ;
#17417=DIRECTION('ref_axis',(0.707106781186549,-1.88044240233301E-14,0.707106781186546)) ;
#17418=DIRECTION('center_axis',(0.922434516585793,0.0559079744467156,-0.3820848871709)) ;
#17419=DIRECTION('ref_axis',(0.386153547971702,-0.13355165491274,0.912715395322624)) ;
#17420=DIRECTION('',(-0.922434516585793,-0.0559079744467156,0.3820848871709)) ;
#17421=DIRECTION('center_axis',(-0.99816831025626,-0.0604981355098033,-6.20703204908959E-17)) ;
#17422=DIRECTION('ref_axis',(9.11766083825151E-17,-2.69321673991429E-15,
1.)) ;
#17423=DIRECTION('center_axis',(-0.99816831025626,-0.0604981355098033,-6.20703204908959E-17)) ;
#17424=DIRECTION('ref_axis',(9.11766083825151E-17,-2.69321673991429E-15,
1.)) ;
#17425=DIRECTION('center_axis',(0.922434516585794,0.0559079744467156,0.382084887170899)) ;
#17426=DIRECTION('ref_axis',(0.386153547971701,-0.133551654912741,-0.912715395322625)) ;
#17427=DIRECTION('',(-0.922434516585794,-0.0559079744467156,-0.382084887170899)) ;
#17428=DIRECTION('center_axis',(-0.705811580947752,-0.0604981355097965,
-0.705811580947687)) ;
#17429=DIRECTION('ref_axis',(0.707106781186514,1.71051325088607E-14,-0.707106781186581)) ;
#17430=DIRECTION('center_axis',(0.382084887170903,0.0559079744467155,0.922434516585792)) ;
#17431=DIRECTION('ref_axis',(0.924127230956646,-0.0231154232803136,-0.381385026201834)) ;
#17432=DIRECTION('',(-0.382084887170903,-0.0559079744467155,-0.922434516585792)) ;
#17433=DIRECTION('center_axis',(1.86210961472694E-16,-0.0604981355098033,
-0.99816831025626)) ;
#17434=DIRECTION('ref_axis',(1.,8.01552601164967E-18,1.28248416186395E-16)) ;
#17435=DIRECTION('center_axis',(-0.382084887170906,0.0559079744467155,0.922434516585791)) ;
#17436=DIRECTION('ref_axis',(0.924127230956645,0.0231154232803138,0.381385026201837)) ;
#17437=DIRECTION('',(0.382084887170905,-0.0559079744467155,-0.922434516585791)) ;
#17438=DIRECTION('center_axis',(0.705811580947719,-0.0604981355097965,-0.70581158094772)) ;
#17439=DIRECTION('ref_axis',(0.707106781186549,1.90609208557029E-14,0.707106781186546)) ;
#17440=DIRECTION('center_axis',(-0.922434516585792,0.0559079744467155,0.382084887170904)) ;
#17441=DIRECTION('ref_axis',(0.386153547971707,0.133551654912738,0.912715395322623)) ;
#17442=DIRECTION('',(0.922434516585791,-0.0559079744467155,-0.382084887170904)) ;
#17443=DIRECTION('center_axis',(0.99816831025626,-0.0604981355098033,-3.28335275692119E-14)) ;
#17444=DIRECTION('ref_axis',(3.28937148703078E-14,4.16807352605788E-16,
1.)) ;
#17445=DIRECTION('center_axis',(0.99816831025626,-0.0604981355098033,-3.28335275692119E-14)) ;
#17446=DIRECTION('ref_axis',(3.28937148703078E-14,4.16807352605788E-16,
1.)) ;
#17447=DIRECTION('center_axis',(-0.922434516585791,0.0559079744467157,-0.382084887170905)) ;
#17448=DIRECTION('ref_axis',(0.386153547971708,0.133551654912738,-0.912715395322622)) ;
#17449=DIRECTION('',(0.922434516585791,-0.0559079744467157,0.382084887170906)) ;
#17450=DIRECTION('center_axis',(0.70581158094776,-0.0604981355097965,0.705811580947679)) ;
#17451=DIRECTION('ref_axis',(0.707106781186506,-1.64959525319754E-14,-0.707106781186589)) ;
#17452=DIRECTION('center_axis',(0.70581158094776,-0.0604981355097965,0.705811580947679)) ;
#17453=DIRECTION('ref_axis',(0.707106781186506,-1.64959525319754E-14,-0.707106781186589)) ;
#17454=DIRECTION('center_axis',(0.70581158094776,-0.0604981355097965,0.705811580947679)) ;
#17455=DIRECTION('ref_axis',(0.707106781186506,-1.64959525319754E-14,-0.707106781186589)) ;
#17456=DIRECTION('center_axis',(-0.382084887170906,0.0559079744467155,-0.922434516585791)) ;
#17457=DIRECTION('ref_axis',(0.924127230956645,0.0231154232803138,-0.381385026201837)) ;
#17458=DIRECTION('',(0.382084887170905,-0.0559079744467155,0.922434516585791)) ;
#17459=DIRECTION('center_axis',(0.382084887170906,-0.0559079744467155,0.922434516585791)) ;
#17460=DIRECTION('ref_axis',(0.924127230956645,0.0231154232803138,-0.381385026201837)) ;
#17461=DIRECTION('center_axis',(0.382084887170906,-0.0559079744467155,0.922434516585791)) ;
#17462=DIRECTION('ref_axis',(-0.924127230956645,-0.0231154232803138,0.381385026201837)) ;
#21209=CARTESIAN_POINT('',(0.,0.,0.)) ;
#21210=CARTESIAN_POINT('Origin',(-5.94713813917601,0.815,9.0943294517364)) ;
#21211=CARTESIAN_POINT('',(-5.9449992070826,0.765091584487187,9.092190519643)) ;
#21212=CARTESIAN_POINT('',(-5.94927707126941,0.864908415512813,9.09646838382981)) ;
#21213=CARTESIAN_POINT('Origin',(-5.94713813917601,0.815,9.0943294517364)) ;
#21214=CARTESIAN_POINT('Origin',(-5.94713813917601,0.815,9.0943294517364)) ;
#21215=CARTESIAN_POINT('Origin',(-6.1946255125913,0.8,9.19684207832111)) ;
#21216=CARTESIAN_POINT('',(-6.19160060581581,0.750091584487187,9.19684207832111)) ;
#21217=CARTESIAN_POINT('',(-6.19765041936679,0.849908415512813,9.19684207832111)) ;
#21218=CARTESIAN_POINT('Origin',(-6.1946255125913,0.8,9.19684207832111)) ;
#21219=CARTESIAN_POINT('',(-6.21393318998988,0.806677582745637,9.24247784808724)) ;
#21220=CARTESIAN_POINT('Origin',(-6.1946255125913,0.8,9.19684207832111)) ;
#21221=CARTESIAN_POINT('',(-6.21375968420955,0.8,9.24303605494667)) ;
#21222=CARTESIAN_POINT('Origin',(-6.1946255125913,0.8,9.19684207832111)) ;
#21223=CARTESIAN_POINT('',(-6.1946255125913,0.8,9.24684207832111)) ;
#21224=CARTESIAN_POINT('Origin',(-6.1946255125913,0.8,9.19684207832111)) ;
#21225=CARTESIAN_POINT('Origin',(-6.1946255125913,0.8,9.19684207832111)) ;
#21226=CARTESIAN_POINT('Origin',(-6.44211288600659,0.785,9.0943294517364)) ;
#21227=CARTESIAN_POINT('',(-6.43997395391319,0.735091584487187,9.09646838382981)) ;
#21228=CARTESIAN_POINT('',(-6.46142056340518,0.791677582745637,9.13996522150253)) ;
#21229=CARTESIAN_POINT('Origin',(-6.44211288600659,0.785,9.0943294517364)) ;
#21230=CARTESIAN_POINT('',(-6.4442518181,0.834908415512813,9.092190519643)) ;
#21231=CARTESIAN_POINT('Origin',(-6.44211288600659,0.785,9.0943294517364)) ;
#21232=CARTESIAN_POINT('',(-6.48831924755442,0.786155771164016,9.11339870304649)) ;
#21233=CARTESIAN_POINT('Origin',(-6.44211288600659,0.785,9.0943294517364)) ;
#21234=CARTESIAN_POINT('Origin',(-6.44211288600659,0.785,9.0943294517364)) ;
#21235=CARTESIAN_POINT('Origin',(-6.5446255125913,0.77,8.84684207832111)) ;
#21236=CARTESIAN_POINT('',(-6.5446255125913,0.720091584487187,8.8498669850966)) ;
#21237=CARTESIAN_POINT('',(-6.59083187413913,0.771155771164016,8.8659113296312)) ;
#21238=CARTESIAN_POINT('Origin',(-6.5446255125913,0.77,8.84684207832111)) ;
#21239=CARTESIAN_POINT('',(-6.5446255125913,0.819908415512813,8.84381717154562)) ;
#21240=CARTESIAN_POINT('Origin',(-6.5446255125913,0.77,8.84684207832111)) ;
#21241=CARTESIAN_POINT('',(-6.59083187413913,0.768844228835984,8.82777282701102)) ;
#21242=CARTESIAN_POINT('Origin',(-6.5446255125913,0.77,8.84684207832111)) ;
#21243=CARTESIAN_POINT('Origin',(-6.5446255125913,0.77,8.84684207832111)) ;
#21244=CARTESIAN_POINT('Origin',(-6.44211288600659,0.755,8.59935470490582)) ;
#21245=CARTESIAN_POINT('',(-6.4442518181,0.705091584487187,8.60149363699922)) ;
#21246=CARTESIAN_POINT('',(-6.48831924755442,0.753844228835984,8.58028545359573)) ;
#21247=CARTESIAN_POINT('Origin',(-6.44211288600659,0.755,8.59935470490582)) ;
#21248=CARTESIAN_POINT('',(-6.43997395391318,0.804908415512813,8.59721577281241)) ;
#21249=CARTESIAN_POINT('Origin',(-6.44211288600659,0.755,8.59935470490582)) ;
#21250=CARTESIAN_POINT('',(-6.46142056340518,0.748322417254363,8.55371893513969)) ;
#21251=CARTESIAN_POINT('Origin',(-6.44211288600659,0.755,8.59935470490582)) ;
#21252=CARTESIAN_POINT('Origin',(-6.44211288600659,0.755,8.59935470490582)) ;
#21253=CARTESIAN_POINT('Origin',(-6.1946255125913,0.74,8.49684207832111)) ;
#21254=CARTESIAN_POINT('',(-6.19765041936679,0.690091584487187,8.49684207832111)) ;
#21255=CARTESIAN_POINT('',(-6.21393318998988,0.733322417254363,8.45120630855498)) ;
#21256=CARTESIAN_POINT('Origin',(-6.1946255125913,0.74,8.49684207832111)) ;
#21257=CARTESIAN_POINT('',(-6.21375968420955,0.74,8.45064810169555)) ;
#21258=CARTESIAN_POINT('Origin',(-6.1946255125913,0.74,8.49684207832111)) ;
#21259=CARTESIAN_POINT('',(-6.1946255125913,0.74,8.44684207832111)) ;
#21260=CARTESIAN_POINT('Origin',(-6.1946255125913,0.74,8.49684207832111)) ;
#21261=CARTESIAN_POINT('',(-6.19160060581581,0.789908415512813,8.49684207832111)) ;
#21262=CARTESIAN_POINT('Origin',(-6.1946255125913,0.74,8.49684207832111)) ;
#21263=CARTESIAN_POINT('Origin',(-6.1946255125913,0.74,8.49684207832111)) ;
#21264=CARTESIAN_POINT('Origin',(-5.94713813917601,0.725,8.59935470490582)) ;
#21265=CARTESIAN_POINT('',(-5.94927707126941,0.675091584487187,8.59721577281241)) ;
#21266=CARTESIAN_POINT('',(-5.9449992070826,0.774908415512813,8.60149363699922)) ;
#21267=CARTESIAN_POINT('Origin',(-5.94713813917601,0.725,8.59935470490582)) ;
#21268=CARTESIAN_POINT('Origin',(-5.94713813917601,0.725,8.59935470490582)) ;
#21269=CARTESIAN_POINT('Origin',(-5.8446255125913,0.71,8.84684207832111)) ;
#21270=CARTESIAN_POINT('',(-5.8446255125913,0.660091584487187,8.84381717154562)) ;
#21271=CARTESIAN_POINT('',(-5.8446255125913,0.759908415512813,8.8498669850966)) ;
#21272=CARTESIAN_POINT('Origin',(-5.8446255125913,0.71,8.84684207832111)) ;
#21273=CARTESIAN_POINT('Origin',(-5.8446255125913,0.71,8.84684207832111)) ;
#21274=CARTESIAN_POINT('Origin',(-5.94713813917601,0.695,9.0943294517364)) ;
#21275=CARTESIAN_POINT('',(-5.9449992070826,0.645091584487187,9.092190519643)) ;
#21276=CARTESIAN_POINT('',(-5.94927707126941,0.744908415512813,9.09646838382981)) ;
#21277=CARTESIAN_POINT('Origin',(-5.94713813917601,0.695,9.0943294517364)) ;
#21278=CARTESIAN_POINT('Origin',(-5.94713813917601,0.695,9.0943294517364)) ;
#21279=CARTESIAN_POINT('Origin',(-6.1946255125913,0.68,9.19684207832111)) ;
#21280=CARTESIAN_POINT('',(-6.19160060581581,0.630091584487187,9.19684207832111)) ;
#21281=CARTESIAN_POINT('',(-6.19765041936679,0.729908415512813,9.19684207832111)) ;
#21282=CARTESIAN_POINT('Origin',(-6.1946255125913,0.68,9.19684207832111)) ;
#21283=CARTESIAN_POINT('',(-6.21393318998988,0.686677582745637,9.24247784808724)) ;
#21284=CARTESIAN_POINT('Origin',(-6.1946255125913,0.68,9.19684207832111)) ;
#21285=CARTESIAN_POINT('',(-6.21375968420955,0.68,9.24303605494667)) ;
#21286=CARTESIAN_POINT('Origin',(-6.1946255125913,0.68,9.19684207832111)) ;
#21287=CARTESIAN_POINT('',(-6.1946255125913,0.68,9.24684207832111)) ;
#21288=CARTESIAN_POINT('Origin',(-6.1946255125913,0.68,9.19684207832111)) ;
#21289=CARTESIAN_POINT('Origin',(-6.1946255125913,0.68,9.19684207832111)) ;
#21290=CARTESIAN_POINT('Origin',(-6.44211288600659,0.665,9.0943294517364)) ;
#21291=CARTESIAN_POINT('',(-6.43997395391319,0.615091584487187,9.09646838382981)) ;
#21292=CARTESIAN_POINT('',(-6.46142056340518,0.671677582745637,9.13996522150253)) ;
#21293=CARTESIAN_POINT('Origin',(-6.44211288600659,0.665,9.0943294517364)) ;
#21294=CARTESIAN_POINT('',(-6.4442518181,0.714908415512813,9.092190519643)) ;
#21295=CARTESIAN_POINT('Origin',(-6.44211288600659,0.665,9.0943294517364)) ;
#21296=CARTESIAN_POINT('',(-6.48831924755442,0.666155771164016,9.11339870304649)) ;
#21297=CARTESIAN_POINT('Origin',(-6.44211288600659,0.665,9.0943294517364)) ;
#21298=CARTESIAN_POINT('Origin',(-6.44211288600659,0.665,9.0943294517364)) ;
#21299=CARTESIAN_POINT('Origin',(-6.5446255125913,0.65,8.84684207832111)) ;
#21300=CARTESIAN_POINT('',(-6.5446255125913,0.600091584487187,8.8498669850966)) ;
#21301=CARTESIAN_POINT('',(-6.59083187413913,0.651155771164016,8.8659113296312)) ;
#21302=CARTESIAN_POINT('Origin',(-6.5446255125913,0.65,8.84684207832111)) ;
#21303=CARTESIAN_POINT('',(-6.5446255125913,0.699908415512813,8.84381717154562)) ;
#21304=CARTESIAN_POINT('Origin',(-6.5446255125913,0.65,8.84684207832111)) ;
#21305=CARTESIAN_POINT('',(-6.59083187413913,0.648844228835984,8.82777282701102)) ;
#21306=CARTESIAN_POINT('Origin',(-6.5446255125913,0.65,8.84684207832111)) ;
#21307=CARTESIAN_POINT('Origin',(-6.5446255125913,0.65,8.84684207832111)) ;
#21308=CARTESIAN_POINT('Origin',(-6.44211288600659,0.635,8.59935470490582)) ;
#21309=CARTESIAN_POINT('',(-6.4442518181,0.585091584487187,8.60149363699922)) ;
#21310=CARTESIAN_POINT('',(-6.48831924755442,0.633844228835984,8.58028545359573)) ;
#21311=CARTESIAN_POINT('Origin',(-6.44211288600659,0.635,8.59935470490582)) ;
#21312=CARTESIAN_POINT('',(-6.43997395391318,0.684908415512813,8.59721577281241)) ;
#21313=CARTESIAN_POINT('Origin',(-6.44211288600659,0.635,8.59935470490582)) ;
#21314=CARTESIAN_POINT('',(-6.46142056340518,0.628322417254363,8.55371893513969)) ;
#21315=CARTESIAN_POINT('Origin',(-6.44211288600659,0.635,8.59935470490582)) ;
#21316=CARTESIAN_POINT('Origin',(-6.44211288600659,0.635,8.59935470490582)) ;
#21317=CARTESIAN_POINT('Origin',(-6.1946255125913,0.62,8.49684207832111)) ;
#21318=CARTESIAN_POINT('',(-6.19765041936679,0.570091584487187,8.49684207832111)) ;
#21319=CARTESIAN_POINT('',(-6.21393318998988,0.613322417254363,8.45120630855498)) ;
#21320=CARTESIAN_POINT('Origin',(-6.1946255125913,0.62,8.49684207832111)) ;
#21321=CARTESIAN_POINT('',(-6.21375968420955,0.62,8.45064810169555)) ;
#21322=CARTESIAN_POINT('Origin',(-6.1946255125913,0.62,8.49684207832111)) ;
#21323=CARTESIAN_POINT('',(-6.1946255125913,0.62,8.44684207832111)) ;
#21324=CARTESIAN_POINT('Origin',(-6.1946255125913,0.62,8.49684207832111)) ;
#21325=CARTESIAN_POINT('',(-6.19160060581581,0.669908415512813,8.49684207832111)) ;
#21326=CARTESIAN_POINT('Origin',(-6.1946255125913,0.62,8.49684207832111)) ;
#21327=CARTESIAN_POINT('Origin',(-6.1946255125913,0.62,8.49684207832111)) ;
#21328=CARTESIAN_POINT('Origin',(-5.94713813917601,0.605,8.59935470490582)) ;
#21329=CARTESIAN_POINT('',(-5.94927707126941,0.555091584487187,8.59721577281241)) ;
#21330=CARTESIAN_POINT('',(-5.9449992070826,0.654908415512813,8.60149363699922)) ;
#21331=CARTESIAN_POINT('Origin',(-5.94713813917601,0.605,8.59935470490582)) ;
#21332=CARTESIAN_POINT('Origin',(-5.94713813917601,0.605,8.59935470490582)) ;
#21333=CARTESIAN_POINT('Origin',(-5.8446255125913,0.59,8.84684207832111)) ;
#21334=CARTESIAN_POINT('',(-5.8446255125913,0.540091584487187,8.84381717154562)) ;
#21335=CARTESIAN_POINT('',(-5.8446255125913,0.639908415512813,8.8498669850966)) ;
#21336=CARTESIAN_POINT('Origin',(-5.8446255125913,0.59,8.84684207832111)) ;
#21337=CARTESIAN_POINT('Origin',(-5.8446255125913,0.59,8.84684207832111)) ;
#21338=CARTESIAN_POINT('Origin',(-5.94713813917601,0.575,9.0943294517364)) ;
#21339=CARTESIAN_POINT('',(-5.9449992070826,0.525091584487187,9.092190519643)) ;
#21340=CARTESIAN_POINT('',(-5.94927707126941,0.624908415512813,9.09646838382981)) ;
#21341=CARTESIAN_POINT('Origin',(-5.94713813917601,0.575,9.0943294517364)) ;
#21342=CARTESIAN_POINT('Origin',(-5.94713813917601,0.575,9.0943294517364)) ;
#21343=CARTESIAN_POINT('Origin',(-6.1946255125913,0.56,9.19684207832111)) ;
#21344=CARTESIAN_POINT('',(-6.19160060581581,0.510091584487187,9.19684207832111)) ;
#21345=CARTESIAN_POINT('',(-6.19765041936679,0.609908415512813,9.19684207832111)) ;
#21346=CARTESIAN_POINT('Origin',(-6.1946255125913,0.56,9.19684207832111)) ;
#21347=CARTESIAN_POINT('',(-6.21393318998988,0.566677582745637,9.24247784808724)) ;
#21348=CARTESIAN_POINT('Origin',(-6.1946255125913,0.56,9.19684207832111)) ;
#21349=CARTESIAN_POINT('',(-6.21375968420955,0.56,9.24303605494667)) ;
#21350=CARTESIAN_POINT('Origin',(-6.1946255125913,0.56,9.19684207832111)) ;
#21351=CARTESIAN_POINT('',(-6.1946255125913,0.56,9.24684207832111)) ;
#21352=CARTESIAN_POINT('Origin',(-6.1946255125913,0.56,9.19684207832111)) ;
#21353=CARTESIAN_POINT('Origin',(-6.1946255125913,0.56,9.19684207832111)) ;
#21354=CARTESIAN_POINT('Origin',(-6.44211288600659,0.545,9.0943294517364)) ;
#21355=CARTESIAN_POINT('',(-6.43997395391318,0.495091584487187,9.09646838382981)) ;
#21356=CARTESIAN_POINT('',(-6.46142056340518,0.551677582745637,9.13996522150253)) ;
#21357=CARTESIAN_POINT('Origin',(-6.44211288600659,0.545,9.0943294517364)) ;
#21358=CARTESIAN_POINT('',(-6.4442518181,0.594908415512813,9.09219051964299)) ;
#21359=CARTESIAN_POINT('Origin',(-6.44211288600659,0.545,9.0943294517364)) ;
#21360=CARTESIAN_POINT('',(-6.48831924755442,0.546155771164016,9.11339870304649)) ;
#21361=CARTESIAN_POINT('Origin',(-6.44211288600659,0.545,9.0943294517364)) ;
#21362=CARTESIAN_POINT('Origin',(-6.44211288600659,0.545,9.0943294517364)) ;
#21363=CARTESIAN_POINT('Origin',(-6.5446255125913,0.53,8.84684207832111)) ;
#21364=CARTESIAN_POINT('',(-6.5446255125913,0.480091584487187,8.8498669850966)) ;
#21365=CARTESIAN_POINT('',(-6.59083187413913,0.531155771164016,8.8659113296312)) ;
#21366=CARTESIAN_POINT('Origin',(-6.5446255125913,0.53,8.84684207832111)) ;
#21367=CARTESIAN_POINT('',(-6.5446255125913,0.579908415512813,8.84381717154562)) ;
#21368=CARTESIAN_POINT('Origin',(-6.5446255125913,0.53,8.84684207832111)) ;
#21369=CARTESIAN_POINT('',(-6.59083187413913,0.528844228835984,8.82777282701102)) ;
#21370=CARTESIAN_POINT('Origin',(-6.5446255125913,0.53,8.84684207832111)) ;
#21371=CARTESIAN_POINT('Origin',(-6.5446255125913,0.53,8.84684207832111)) ;
#21372=CARTESIAN_POINT('Origin',(-6.44211288600659,0.515,8.59935470490582)) ;
#21373=CARTESIAN_POINT('',(-6.4442518181,0.465091584487187,8.60149363699922)) ;
#21374=CARTESIAN_POINT('',(-6.48831924755442,0.513844228835984,8.58028545359573)) ;
#21375=CARTESIAN_POINT('Origin',(-6.44211288600659,0.515,8.59935470490582)) ;
#21376=CARTESIAN_POINT('',(-6.43997395391318,0.564908415512813,8.59721577281241)) ;
#21377=CARTESIAN_POINT('Origin',(-6.44211288600659,0.515,8.59935470490582)) ;
#21378=CARTESIAN_POINT('',(-6.46142056340518,0.508322417254363,8.55371893513969)) ;
#21379=CARTESIAN_POINT('Origin',(-6.44211288600659,0.515,8.59935470490582)) ;
#21380=CARTESIAN_POINT('Origin',(-6.44211288600659,0.515,8.59935470490582)) ;
#21381=CARTESIAN_POINT('Origin',(-6.1946255125913,0.5,8.49684207832111)) ;
#21382=CARTESIAN_POINT('',(-6.19765041936679,0.450091584487187,8.49684207832111)) ;
#21383=CARTESIAN_POINT('',(-6.21393318998988,0.493322417254363,8.45120630855498)) ;
#21384=CARTESIAN_POINT('Origin',(-6.1946255125913,0.5,8.49684207832111)) ;
#21385=CARTESIAN_POINT('',(-6.21375968420955,0.5,8.45064810169555)) ;
#21386=CARTESIAN_POINT('Origin',(-6.1946255125913,0.5,8.49684207832111)) ;
#21387=CARTESIAN_POINT('',(-6.1946255125913,0.5,8.44684207832111)) ;
#21388=CARTESIAN_POINT('Origin',(-6.1946255125913,0.5,8.49684207832111)) ;
#21389=CARTESIAN_POINT('',(-6.19160060581581,0.549908415512813,8.49684207832111)) ;
#21390=CARTESIAN_POINT('Origin',(-6.1946255125913,0.5,8.49684207832111)) ;
#21391=CARTESIAN_POINT('Origin',(-6.1946255125913,0.5,8.49684207832111)) ;
#21392=CARTESIAN_POINT('Origin',(-5.94713813917601,0.485,8.59935470490582)) ;
#21393=CARTESIAN_POINT('',(-5.94927707126941,0.435091584487187,8.59721577281241)) ;
#21394=CARTESIAN_POINT('',(-5.9449992070826,0.534908415512813,8.60149363699922)) ;
#21395=CARTESIAN_POINT('Origin',(-5.94713813917601,0.485,8.59935470490582)) ;
#21396=CARTESIAN_POINT('Origin',(-5.94713813917601,0.485,8.59935470490582)) ;
#21397=CARTESIAN_POINT('Origin',(-5.8446255125913,0.47,8.84684207832111)) ;
#21398=CARTESIAN_POINT('',(-5.8446255125913,0.420091584487187,8.84381717154562)) ;
#21399=CARTESIAN_POINT('',(-5.8446255125913,0.519908415512813,8.8498669850966)) ;
#21400=CARTESIAN_POINT('Origin',(-5.8446255125913,0.47,8.84684207832111)) ;
#21401=CARTESIAN_POINT('Origin',(-5.8446255125913,0.47,8.84684207832111)) ;
#21402=CARTESIAN_POINT('Origin',(-5.94713813917601,0.455,9.0943294517364)) ;
#21403=CARTESIAN_POINT('',(-5.9449992070826,0.405091584487187,9.092190519643)) ;
#21404=CARTESIAN_POINT('',(-5.94927707126941,0.504908415512813,9.09646838382981)) ;
#21405=CARTESIAN_POINT('Origin',(-5.94713813917601,0.455,9.0943294517364)) ;
#21406=CARTESIAN_POINT('Origin',(-5.94713813917601,0.455,9.0943294517364)) ;
#21407=CARTESIAN_POINT('Origin',(-6.1946255125913,0.44,9.19684207832111)) ;
#21408=CARTESIAN_POINT('',(-6.19160060581581,0.390091584487187,9.19684207832111)) ;
#21409=CARTESIAN_POINT('',(-6.19765041936679,0.489908415512813,9.19684207832111)) ;
#21410=CARTESIAN_POINT('Origin',(-6.1946255125913,0.44,9.19684207832111)) ;
#21411=CARTESIAN_POINT('',(-6.21393318998988,0.446677582745637,9.24247784808724)) ;
#21412=CARTESIAN_POINT('Origin',(-6.1946255125913,0.44,9.19684207832111)) ;
#21413=CARTESIAN_POINT('',(-6.21375968420955,0.44,9.24303605494667)) ;
#21414=CARTESIAN_POINT('Origin',(-6.1946255125913,0.44,9.19684207832111)) ;
#21415=CARTESIAN_POINT('',(-6.1946255125913,0.44,9.24684207832111)) ;
#21416=CARTESIAN_POINT('Origin',(-6.1946255125913,0.44,9.19684207832111)) ;
#21417=CARTESIAN_POINT('Origin',(-6.1946255125913,0.44,9.19684207832111)) ;
#21418=CARTESIAN_POINT('Origin',(-6.44211288600659,0.425,9.0943294517364)) ;
#21419=CARTESIAN_POINT('',(-6.43997395391318,0.375091584487187,9.09646838382981)) ;
#21420=CARTESIAN_POINT('',(-6.46142056340518,0.431677582745637,9.13996522150253)) ;
#21421=CARTESIAN_POINT('Origin',(-6.44211288600659,0.425,9.0943294517364)) ;
#21422=CARTESIAN_POINT('',(-6.4442518181,0.474908415512813,9.09219051964299)) ;
#21423=CARTESIAN_POINT('Origin',(-6.44211288600659,0.425,9.0943294517364)) ;
#21424=CARTESIAN_POINT('',(-6.48831924755442,0.426155771164016,9.1133987030465)) ;
#21425=CARTESIAN_POINT('Origin',(-6.44211288600659,0.425,9.0943294517364)) ;
#21426=CARTESIAN_POINT('Origin',(-6.44211288600659,0.425,9.0943294517364)) ;
#21427=CARTESIAN_POINT('Origin',(-6.5446255125913,0.41,8.84684207832111)) ;
#21428=CARTESIAN_POINT('',(-6.5446255125913,0.360091584487187,8.8498669850966)) ;
#21429=CARTESIAN_POINT('',(-6.59083187413913,0.411155771164016,8.8659113296312)) ;
#21430=CARTESIAN_POINT('Origin',(-6.5446255125913,0.41,8.84684207832111)) ;
#21431=CARTESIAN_POINT('',(-6.5446255125913,0.459908415512813,8.84381717154562)) ;
#21432=CARTESIAN_POINT('Origin',(-6.5446255125913,0.41,8.84684207832111)) ;
#21433=CARTESIAN_POINT('',(-6.59083187413913,0.408844228835984,8.82777282701102)) ;
#21434=CARTESIAN_POINT('Origin',(-6.5446255125913,0.41,8.84684207832111)) ;
#21435=CARTESIAN_POINT('Origin',(-6.5446255125913,0.41,8.84684207832111)) ;
#21436=CARTESIAN_POINT('Origin',(-6.44211288600659,0.395,8.59935470490582)) ;
#21437=CARTESIAN_POINT('',(-6.4442518181,0.345091584487187,8.60149363699923)) ;
#21438=CARTESIAN_POINT('',(-6.48831924755442,0.393844228835984,8.58028545359573)) ;
#21439=CARTESIAN_POINT('Origin',(-6.44211288600659,0.395,8.59935470490582)) ;
#21440=CARTESIAN_POINT('',(-6.43997395391318,0.444908415512813,8.59721577281242)) ;
#21441=CARTESIAN_POINT('Origin',(-6.44211288600659,0.395,8.59935470490582)) ;
#21442=CARTESIAN_POINT('',(-6.46142056340518,0.388322417254363,8.55371893513969)) ;
#21443=CARTESIAN_POINT('Origin',(-6.44211288600659,0.395,8.59935470490582)) ;
#21444=CARTESIAN_POINT('Origin',(-6.44211288600659,0.395,8.59935470490582)) ;
#21445=CARTESIAN_POINT('Origin',(-6.1946255125913,0.38,8.49684207832111)) ;
#21446=CARTESIAN_POINT('',(-6.19765041936679,0.330091584487187,8.49684207832111)) ;
#21447=CARTESIAN_POINT('',(-6.21393318998988,0.373322417254363,8.45120630855498)) ;
#21448=CARTESIAN_POINT('Origin',(-6.1946255125913,0.38,8.49684207832111)) ;
#21449=CARTESIAN_POINT('',(-6.21375968420955,0.38,8.45064810169555)) ;
#21450=CARTESIAN_POINT('Origin',(-6.1946255125913,0.38,8.49684207832111)) ;
#21451=CARTESIAN_POINT('',(-6.1946255125913,0.38,8.44684207832111)) ;
#21452=CARTESIAN_POINT('Origin',(-6.1946255125913,0.38,8.49684207832111)) ;
#21453=CARTESIAN_POINT('',(-6.19160060581581,0.429908415512813,8.49684207832111)) ;
#21454=CARTESIAN_POINT('Origin',(-6.1946255125913,0.38,8.49684207832111)) ;
#21455=CARTESIAN_POINT('Origin',(-6.1946255125913,0.38,8.49684207832111)) ;
#21456=CARTESIAN_POINT('Origin',(-5.94713813917601,0.365,8.59935470490582)) ;
#21457=CARTESIAN_POINT('',(-5.94927707126941,0.315091584487187,8.59721577281241)) ;
#21458=CARTESIAN_POINT('',(-5.9449992070826,0.414908415512813,8.60149363699922)) ;
#21459=CARTESIAN_POINT('Origin',(-5.94713813917601,0.365,8.59935470490582)) ;
#21460=CARTESIAN_POINT('Origin',(-5.94713813917601,0.365,8.59935470490582)) ;
#21461=CARTESIAN_POINT('Origin',(-5.89588182588365,0.8225,8.97058576502876)) ;
#21462=CARTESIAN_POINT('',(-5.89083187413913,0.831155771164016,8.82777282701102)) ;
#21463=CARTESIAN_POINT('Origin',(-5.8446255125913,0.83,8.84684207832111)) ;
#21464=CARTESIAN_POINT('',(-5.98545422562987,0.817310303345588,9.05621139128359)) ;
#21465=CARTESIAN_POINT('',(-5.94208818743149,0.823655771164016,8.95151651371867)) ;
#21466=CARTESIAN_POINT('',(-5.98539769271865,0.820528925590979,9.05654380610156)) ;
#21467=CARTESIAN_POINT('Origin',(-5.94713813917601,0.815,9.0943294517364)) ;
#21468=CARTESIAN_POINT('Origin',(-5.94713813917601,0.815,9.0943294517364)) ;
#21469=CARTESIAN_POINT('Origin',(-5.94713813917601,0.815,9.0943294517364)) ;
#21470=CARTESIAN_POINT('Origin',(-5.8446255125913,0.83,8.84684207832111)) ;
#21471=CARTESIAN_POINT('Origin',(-6.07088182588365,0.8075,9.14558576502876)) ;
#21472=CARTESIAN_POINT('',(-6.1950994204991,0.807819081556115,9.14340510580129)) ;
#21473=CARTESIAN_POINT('',(-6.09018950328224,0.814177582745637,9.09994999526262)) ;
#21474=CARTESIAN_POINT('Origin',(-6.1946255125913,0.8,9.19684207832111)) ;
#21475=CARTESIAN_POINT('Origin',(-6.1946255125913,0.8,9.19684207832111)) ;
#21476=CARTESIAN_POINT('Origin',(-6.31836919929895,0.7925,9.14558576502876)) ;
#21477=CARTESIAN_POINT('',(-6.33767687669753,0.799177582745637,9.19122153479489)) ;
#21478=CARTESIAN_POINT('Origin',(-6.44211288600659,0.785,9.0943294517364)) ;
#21479=CARTESIAN_POINT('Origin',(-6.49336919929894,0.7775,8.97058576502876)) ;
#21480=CARTESIAN_POINT('',(-6.53957556084678,0.778655771164016,8.98965501633885)) ;
#21481=CARTESIAN_POINT('Origin',(-6.5446255125913,0.77,8.84684207832111)) ;
#21482=CARTESIAN_POINT('Origin',(-6.49336919929894,0.7625,8.72309839161347)) ;
#21483=CARTESIAN_POINT('',(-6.53957556084678,0.761344228835984,8.70402914030337)) ;
#21484=CARTESIAN_POINT('Origin',(-6.44211288600659,0.755,8.59935470490582)) ;
#21485=CARTESIAN_POINT('Origin',(-6.31836919929894,0.7475,8.54809839161346)) ;
#21486=CARTESIAN_POINT('',(-6.33767687669753,0.740822417254363,8.50246262184733)) ;
#21487=CARTESIAN_POINT('',(-6.1950994204991,0.732180918443886,8.55027905084093)) ;
#21488=CARTESIAN_POINT('Origin',(-6.1946255125913,0.74,8.49684207832111)) ;
#21489=CARTESIAN_POINT('Origin',(-6.1946255125913,0.74,8.49684207832111)) ;
#21490=CARTESIAN_POINT('Origin',(-6.07088182588365,0.7325,8.54809839161346)) ;
#21491=CARTESIAN_POINT('',(-5.98539769271865,0.719471074409021,8.63714035054067)) ;
#21492=CARTESIAN_POINT('',(-6.09018950328224,0.725822417254363,8.5937341613796)) ;
#21493=CARTESIAN_POINT('',(-5.98545422562987,0.722689696654412,8.63747276535863)) ;
#21494=CARTESIAN_POINT('Origin',(-5.94713813917601,0.725,8.59935470490582)) ;
#21495=CARTESIAN_POINT('Origin',(-5.94713813917601,0.725,8.59935470490582)) ;
#21496=CARTESIAN_POINT('Origin',(-5.94713813917601,0.725,8.59935470490582)) ;
#21497=CARTESIAN_POINT('Origin',(-5.89588182588365,0.7175,8.72309839161347)) ;
#21498=CARTESIAN_POINT('',(-5.89873061665607,0.71,8.84684207832111)) ;
#21499=CARTESIAN_POINT('',(-5.94208818743149,0.716344228835984,8.74216764292356)) ;
#21500=CARTESIAN_POINT('Origin',(-5.8446255125913,0.71,8.84684207832111)) ;
#21501=CARTESIAN_POINT('Origin',(-5.8446255125913,0.71,8.84684207832111)) ;
#21502=CARTESIAN_POINT('Origin',(-5.89588182588365,0.7025,8.97058576502876)) ;
#21503=CARTESIAN_POINT('',(-5.98545422562987,0.697310303345588,9.05621139128359)) ;
#21504=CARTESIAN_POINT('',(-5.94208818743149,0.703655771164016,8.95151651371867)) ;
#21505=CARTESIAN_POINT('',(-5.98539769271865,0.700528925590979,9.05654380610155)) ;
#21506=CARTESIAN_POINT('Origin',(-5.94713813917601,0.695,9.0943294517364)) ;
#21507=CARTESIAN_POINT('Origin',(-5.94713813917601,0.695,9.0943294517364)) ;
#21508=CARTESIAN_POINT('Origin',(-5.94713813917601,0.695,9.0943294517364)) ;
#21509=CARTESIAN_POINT('Origin',(-6.07088182588365,0.6875,9.14558576502876)) ;
#21510=CARTESIAN_POINT('',(-6.1950994204991,0.687819081556115,9.14340510580129)) ;
#21511=CARTESIAN_POINT('',(-6.09018950328224,0.694177582745637,9.09994999526262)) ;
#21512=CARTESIAN_POINT('Origin',(-6.1946255125913,0.68,9.19684207832111)) ;
#21513=CARTESIAN_POINT('Origin',(-6.1946255125913,0.68,9.19684207832111)) ;
#21514=CARTESIAN_POINT('Origin',(-6.31836919929895,0.6725,9.14558576502876)) ;
#21515=CARTESIAN_POINT('',(-6.33767687669753,0.679177582745637,9.19122153479489)) ;
#21516=CARTESIAN_POINT('Origin',(-6.44211288600659,0.665,9.0943294517364)) ;
#21517=CARTESIAN_POINT('Origin',(-6.49336919929894,0.6575,8.97058576502876)) ;
#21518=CARTESIAN_POINT('',(-6.53957556084678,0.658655771164016,8.98965501633885)) ;
#21519=CARTESIAN_POINT('Origin',(-6.5446255125913,0.65,8.84684207832111)) ;
#21520=CARTESIAN_POINT('Origin',(-6.49336919929894,0.6425,8.72309839161347)) ;
#21521=CARTESIAN_POINT('',(-6.53957556084678,0.641344228835984,8.70402914030337)) ;
#21522=CARTESIAN_POINT('Origin',(-6.44211288600659,0.635,8.59935470490582)) ;
#21523=CARTESIAN_POINT('Origin',(-6.31836919929894,0.6275,8.54809839161346)) ;
#21524=CARTESIAN_POINT('',(-6.33767687669753,0.620822417254363,8.50246262184733)) ;
#21525=CARTESIAN_POINT('',(-6.1950994204991,0.612180918443886,8.55027905084093)) ;
#21526=CARTESIAN_POINT('Origin',(-6.1946255125913,0.62,8.49684207832111)) ;
#21527=CARTESIAN_POINT('Origin',(-6.1946255125913,0.62,8.49684207832111)) ;
#21528=CARTESIAN_POINT('Origin',(-6.07088182588365,0.6125,8.54809839161346)) ;
#21529=CARTESIAN_POINT('',(-5.98539769271865,0.599471074409021,8.63714035054067)) ;
#21530=CARTESIAN_POINT('',(-6.09018950328224,0.605822417254363,8.5937341613796)) ;
#21531=CARTESIAN_POINT('',(-5.98545422562987,0.602689696654412,8.63747276535863)) ;
#21532=CARTESIAN_POINT('Origin',(-5.94713813917601,0.605,8.59935470490582)) ;
#21533=CARTESIAN_POINT('Origin',(-5.94713813917601,0.605,8.59935470490582)) ;
#21534=CARTESIAN_POINT('Origin',(-5.94713813917601,0.605,8.59935470490582)) ;
#21535=CARTESIAN_POINT('Origin',(-5.89588182588365,0.5975,8.72309839161347)) ;
#21536=CARTESIAN_POINT('',(-5.89873061665607,0.59,8.84684207832111)) ;
#21537=CARTESIAN_POINT('',(-5.94208818743149,0.596344228835984,8.74216764292356)) ;
#21538=CARTESIAN_POINT('Origin',(-5.8446255125913,0.59,8.84684207832111)) ;
#21539=CARTESIAN_POINT('Origin',(-5.8446255125913,0.59,8.84684207832111)) ;
#21540=CARTESIAN_POINT('Origin',(-5.89588182588365,0.5825,8.97058576502876)) ;
#21541=CARTESIAN_POINT('',(-5.98545422562987,0.577310303345588,9.05621139128359)) ;
#21542=CARTESIAN_POINT('',(-5.94208818743149,0.583655771164016,8.95151651371867)) ;
#21543=CARTESIAN_POINT('',(-5.98539769271865,0.58052892559098,9.05654380610155)) ;
#21544=CARTESIAN_POINT('Origin',(-5.94713813917601,0.575,9.0943294517364)) ;
#21545=CARTESIAN_POINT('Origin',(-5.94713813917601,0.575,9.0943294517364)) ;
#21546=CARTESIAN_POINT('Origin',(-5.94713813917601,0.575,9.0943294517364)) ;
#21547=CARTESIAN_POINT('Origin',(-6.07088182588365,0.5675,9.14558576502876)) ;
#21548=CARTESIAN_POINT('',(-6.1950994204991,0.567819081556115,9.14340510580128)) ;
#21549=CARTESIAN_POINT('',(-6.09018950328224,0.574177582745637,9.09994999526262)) ;
#21550=CARTESIAN_POINT('Origin',(-6.1946255125913,0.56,9.19684207832111)) ;
#21551=CARTESIAN_POINT('Origin',(-6.1946255125913,0.56,9.19684207832111)) ;
#21552=CARTESIAN_POINT('Origin',(-6.31836919929894,0.5525,9.14558576502876)) ;
#21553=CARTESIAN_POINT('',(-6.33767687669753,0.559177582745637,9.19122153479489)) ;
#21554=CARTESIAN_POINT('Origin',(-6.44211288600659,0.545,9.0943294517364)) ;
#21555=CARTESIAN_POINT('Origin',(-6.49336919929894,0.5375,8.97058576502876)) ;
#21556=CARTESIAN_POINT('',(-6.53957556084678,0.538655771164016,8.98965501633885)) ;
#21557=CARTESIAN_POINT('Origin',(-6.5446255125913,0.53,8.84684207832111)) ;
#21558=CARTESIAN_POINT('Origin',(-6.49336919929894,0.5225,8.72309839161347)) ;
#21559=CARTESIAN_POINT('',(-6.53957556084678,0.521344228835984,8.70402914030337)) ;
#21560=CARTESIAN_POINT('Origin',(-6.44211288600659,0.515,8.59935470490582)) ;
#21561=CARTESIAN_POINT('Origin',(-6.31836919929894,0.5075,8.54809839161346)) ;
#21562=CARTESIAN_POINT('',(-6.33767687669753,0.500822417254363,8.50246262184733)) ;
#21563=CARTESIAN_POINT('',(-6.1950994204991,0.492180918443886,8.55027905084093)) ;
#21564=CARTESIAN_POINT('Origin',(-6.1946255125913,0.5,8.49684207832111)) ;
#21565=CARTESIAN_POINT('Origin',(-6.1946255125913,0.5,8.49684207832111)) ;
#21566=CARTESIAN_POINT('Origin',(-6.07088182588365,0.4925,8.54809839161346)) ;
#21567=CARTESIAN_POINT('',(-5.98539769271865,0.47947107440902,8.63714035054067)) ;
#21568=CARTESIAN_POINT('',(-6.09018950328224,0.485822417254363,8.5937341613796)) ;
#21569=CARTESIAN_POINT('',(-5.98545422562987,0.482689696654412,8.63747276535863)) ;
#21570=CARTESIAN_POINT('Origin',(-5.94713813917601,0.485,8.59935470490582)) ;
#21571=CARTESIAN_POINT('Origin',(-5.94713813917601,0.485,8.59935470490582)) ;
#21572=CARTESIAN_POINT('Origin',(-5.94713813917601,0.485,8.59935470490582)) ;
#21573=CARTESIAN_POINT('Origin',(-5.89588182588365,0.4775,8.72309839161347)) ;
#21574=CARTESIAN_POINT('',(-5.89873061665607,0.47,8.84684207832111)) ;
#21575=CARTESIAN_POINT('',(-5.94208818743149,0.476344228835984,8.74216764292356)) ;
#21576=CARTESIAN_POINT('Origin',(-5.8446255125913,0.47,8.84684207832111)) ;
#21577=CARTESIAN_POINT('Origin',(-5.8446255125913,0.47,8.84684207832111)) ;
#21578=CARTESIAN_POINT('Origin',(-5.89588182588365,0.4625,8.97058576502876)) ;
#21579=CARTESIAN_POINT('',(-5.98545422562987,0.457310303345588,9.05621139128359)) ;
#21580=CARTESIAN_POINT('',(-5.94208818743149,0.463655771164016,8.95151651371867)) ;
#21581=CARTESIAN_POINT('',(-5.98539769271865,0.46052892559098,9.05654380610155)) ;
#21582=CARTESIAN_POINT('Origin',(-5.94713813917601,0.455,9.0943294517364)) ;
#21583=CARTESIAN_POINT('Origin',(-5.94713813917601,0.455,9.0943294517364)) ;
#21584=CARTESIAN_POINT('Origin',(-5.94713813917601,0.455,9.0943294517364)) ;
#21585=CARTESIAN_POINT('Origin',(-6.07088182588365,0.4475,9.14558576502876)) ;
#21586=CARTESIAN_POINT('',(-6.1950994204991,0.447819081556115,9.14340510580128)) ;
#21587=CARTESIAN_POINT('',(-6.09018950328224,0.454177582745637,9.09994999526262)) ;
#21588=CARTESIAN_POINT('Origin',(-6.1946255125913,0.44,9.19684207832111)) ;
#21589=CARTESIAN_POINT('Origin',(-6.1946255125913,0.44,9.19684207832111)) ;
#21590=CARTESIAN_POINT('Origin',(-6.31836919929894,0.4325,9.14558576502876)) ;
#21591=CARTESIAN_POINT('',(-6.33767687669753,0.439177582745637,9.19122153479489)) ;
#21592=CARTESIAN_POINT('Origin',(-6.44211288600659,0.425,9.0943294517364)) ;
#21593=CARTESIAN_POINT('Origin',(-6.49336919929894,0.4175,8.97058576502876)) ;
#21594=CARTESIAN_POINT('',(-6.53957556084678,0.418655771164016,8.98965501633885)) ;
#21595=CARTESIAN_POINT('Origin',(-6.5446255125913,0.41,8.84684207832111)) ;
#21596=CARTESIAN_POINT('Origin',(-6.49336919929894,0.4025,8.72309839161347)) ;
#21597=CARTESIAN_POINT('',(-6.53957556084678,0.401344228835984,8.70402914030337)) ;
#21598=CARTESIAN_POINT('Origin',(-6.44211288600659,0.395,8.59935470490582)) ;
#21599=CARTESIAN_POINT('Origin',(-6.31836919929894,0.3875,8.54809839161346)) ;
#21600=CARTESIAN_POINT('',(-6.33767687669753,0.380822417254363,8.50246262184733)) ;
#21601=CARTESIAN_POINT('',(-6.1950994204991,0.372180918443886,8.55027905084093)) ;
#21602=CARTESIAN_POINT('Origin',(-6.1946255125913,0.38,8.49684207832111)) ;
#21603=CARTESIAN_POINT('Origin',(-6.1946255125913,0.38,8.49684207832111)) ;
#21604=CARTESIAN_POINT('Origin',(-6.07088182588365,0.3725,8.54809839161346)) ;
#21605=CARTESIAN_POINT('',(-5.98539769271865,0.35947107440902,8.63714035054067)) ;
#21606=CARTESIAN_POINT('',(-6.09018950328224,0.365822417254363,8.5937341613796)) ;
#21607=CARTESIAN_POINT('',(-5.98545422562987,0.362689696654412,8.63747276535863)) ;
#21608=CARTESIAN_POINT('Origin',(-5.94713813917601,0.365,8.59935470490582)) ;
#21609=CARTESIAN_POINT('Origin',(-5.94713813917601,0.365,8.59935470490582)) ;
#21610=CARTESIAN_POINT('Origin',(-5.94713813917601,0.365,8.59935470490582)) ;
#21611=CARTESIAN_POINT('Origin',(-5.89588182588365,0.3575,8.72309839161347)) ;
#21612=CARTESIAN_POINT('',(-5.89083187413913,0.348844228835984,8.8659113296312)) ;
#21613=CARTESIAN_POINT('',(-5.94208818743149,0.356344228835984,8.74216764292356)) ;
#21614=CARTESIAN_POINT('Origin',(-5.8446255125913,0.35,8.84684207832111)) ;
#21615=CARTESIAN_POINT('Origin',(-5.8446255125913,0.35,8.84684207832111)) ;
#24551=UNCERTAINTY_MEASURE_WITH_UNIT(LENGTH_MEASURE(0.001),#24629,
'DISTANCE_ACCURACY_VALUE',
'Maximum model space distance between geometric entities at asserted c
onnectivities') ;
#24580=UNCERTAINTY_MEASURE_WITH_UNIT(LENGTH_MEASURE(0.001),#24629,
'DISTANCE_ACCURACY_VALUE',
'Maximum model space distance between geometric entities at asserted c
onnectivities') ;
#24599=(
GEOMETRIC_REPRESENTATION_CONTEXT(3)
GLOBAL_UNCERTAINTY_ASSIGNED_CONTEXT((#24551))
GLOBAL_UNIT_ASSIGNED_CONTEXT((#24629,#24631,#24632))
REPRESENTATION_CONTEXT('','3D')
) ;
#24628=(
GEOMETRIC_REPRESENTATION_CONTEXT(3)
GLOBAL_UNCERTAINTY_ASSIGNED_CONTEXT((#24580))
GLOBAL_UNIT_ASSIGNED_CONTEXT((#24629,#24631,#24632))
REPRESENTATION_CONTEXT('','3D')
) ;
#24629=(
LENGTH_UNIT()
NAMED_UNIT(*)
SI_UNIT(.CENTI.,.METRE.)
) ;
#24631=(
NAMED_UNIT(*)
PLANE_ANGLE_UNIT()
SI_UNIT($,.RADIAN.)
) ;
#24632=(
NAMED_UNIT(*)
SI_UNIT($,.STERADIAN.)
SOLID_ANGLE_UNIT()
) ;
#24651=SHAPE_DEFINITION_REPRESENTATION(#24698,#24809) ;
#24698=PRODUCT_DEFINITION_SHAPE('',$,#24857) ;
#24809=SHAPE_REPRESENTATION('',(#14259),#24599) ;
#24838=PRODUCT_DEFINITION_CONTEXT('part definition',#24981,'design') ;
#24857=PRODUCT_DEFINITION('EJECTOR_TORSION_SPRING',
'EJECTOR_TORSION_SPRING',#24904,#24838) ;
#24904=PRODUCT_DEFINITION_FORMATION('',$,#25001) ;
#24981=APPLICATION_CONTEXT(
'Core Data for Automotive Mechanical Design Process') ;
#24982=PRODUCT_CONTEXT('part definition',#24981,'mechanical') ;
#25001=PRODUCT('EJECTOR_TORSION_SPRING','EJECTOR_TORSION_SPRING',$,(#24982)) ;
#25030=PRESENTATION_STYLE_ASSIGNMENT((#25040)) ;
#25040=SURFACE_STYLE_USAGE(.BOTH.,#25050) ;
#25050=SURFACE_SIDE_STYLE('',(#25060)) ;
#25060=SURFACE_STYLE_FILL_AREA(#25070) ;
#25070=FILL_AREA_STYLE('Steel - Satin',(#25080)) ;
#25080=FILL_AREA_STYLE_COLOUR('Steel - Satin',#25090) ;
#25090=COLOUR_RGB('Steel - Satin', 0.66274510, 0.83137255, 0.94901961) ;
ENDSEC;
END-ISO-10303-21;
